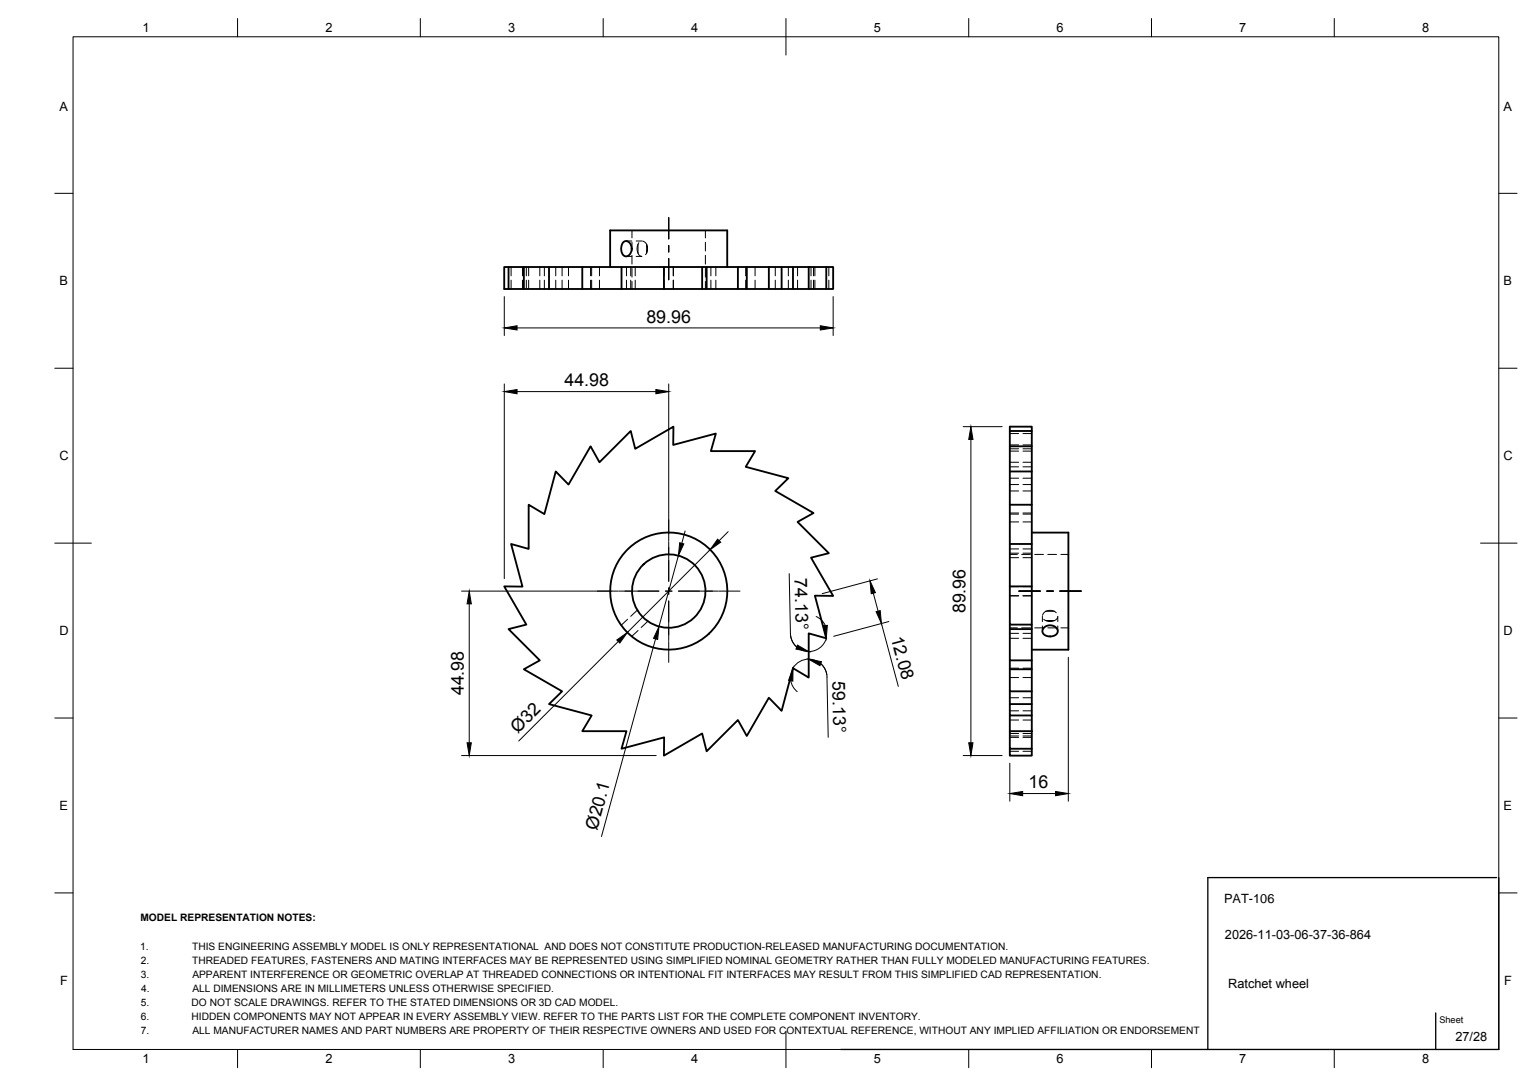
ISO-10303-21;
HEADER;
/* Generated by software containing ST-Developer
 * from STEP Tools, Inc. (www.steptools.com) 
 */

FILE_DESCRIPTION(
/* description */ ('Torsion-spring ratchet demonstrator'),
/* implementation_level */ '2;1');

FILE_NAME(
/* name */ 'Ratchet wheel.step',
/* time_stamp */ '2026-10-29T17:29:17-07:00',
/* author */ (''),
/* organization */ (''),
/* preprocessor_version */ 'ST-DEVELOPER v20.2',
/* originating_system */ 'Autodesk Translation Framework v15.17.0.0',
/* authorisation */ '');

FILE_SCHEMA (('AUTOMOTIVE_DESIGN { 1 0 10303 214 3 1 1 }'));
ENDSEC;

DATA;
#10=MECHANICAL_DESIGN_GEOMETRIC_PRESENTATION_REPRESENTATION('',(#312),#11258);
#231=B_SPLINE_CURVE_WITH_KNOTS('',3,(#10681,#10682,#10683,#10684,#10685,
#10686,#10687,#10688,#10689,#10690,#10691,#10692,#10693,#10694),
 .UNSPECIFIED.,.F.,.F.,(4,2,2,2,2,2,4),(0.75600573798702,0.793568827564647,
0.872922520054201,0.952276212543756,1.03162990503331,1.11098359752287,1.14854668710049),
 .UNSPECIFIED.);
#232=B_SPLINE_CURVE_WITH_KNOTS('',3,(#10700,#10701,#10702,#10703,#10704,
#10705,#10706,#10707,#10708,#10709,#10710,#10711,#10712,#10713,#10714,#10715,
#10716,#10717),.UNSPECIFIED.,.F.,.F.,(4,2,2,2,2,2,2,2,4),(0.,0.0792028026112439,
0.158405605222488,0.237607602356377,0.316809599490267,0.396011596624156,
0.475213593758045,0.554416396369289,0.633619198980533),.UNSPECIFIED.);
#233=B_SPLINE_CURVE_WITH_KNOTS('',3,(#10718,#10719,#10720,#10721,#10722,
#10723,#10724,#10725,#10726,#10727,#10728,#10729,#10730,#10731,#10732,#10733,
#10734,#10735),.UNSPECIFIED.,.F.,.F.,(4,2,2,2,2,2,2,2,4),(0.633619198980533,
0.712822001591777,0.792024804203021,0.87122680133691,0.950428798470799,
1.02963079560469,1.10883279273858,1.18803559534982,1.26723839796107),
 .UNSPECIFIED.);
#234=B_SPLINE_CURVE_WITH_KNOTS('',3,(#10738,#10739,#10740,#10741,#10742,
#10743,#10744,#10745,#10746,#10747,#10748,#10749,#10750,#10751),
 .UNSPECIFIED.,.F.,.F.,(4,2,2,2,2,2,4),(0.121154929624516,0.158718019202143,
0.238071711691697,0.317425404181252,0.396779096670807,0.476132789160362,
0.513695878737989),.UNSPECIFIED.);
#256=SHAPE_REPRESENTATION_RELATIONSHIP('SRR','None',#11384,#280);
#280=ADVANCED_BREP_SHAPE_REPRESENTATION('',(#342),#11254);
#312=STYLED_ITEM('',(#11577),#342);
#342=MANIFOLD_SOLID_BREP('Body1',#5185);
#429=FACE_BOUND('',#1237,.T.);
#430=FACE_BOUND('',#1239,.T.);
#431=FACE_BOUND('',#1241,.T.);
#432=FACE_BOUND('',#1291,.T.);
#433=FACE_BOUND('',#1293,.T.);
#549=PLANE('',#5948);
#550=PLANE('',#5953);
#551=PLANE('',#5957);
#552=PLANE('',#5961);
#553=PLANE('',#5962);
#554=PLANE('',#5963);
#555=PLANE('',#5964);
#556=PLANE('',#5965);
#557=PLANE('',#5966);
#558=PLANE('',#5967);
#559=PLANE('',#5968);
#560=PLANE('',#5969);
#561=PLANE('',#5970);
#562=PLANE('',#5971);
#563=PLANE('',#5972);
#564=PLANE('',#5973);
#565=PLANE('',#5974);
#566=PLANE('',#5975);
#567=PLANE('',#5976);
#568=PLANE('',#5977);
#569=PLANE('',#5978);
#570=PLANE('',#5979);
#571=PLANE('',#5980);
#572=PLANE('',#5981);
#573=PLANE('',#5982);
#574=PLANE('',#5983);
#575=PLANE('',#5984);
#576=PLANE('',#5985);
#577=PLANE('',#5986);
#578=PLANE('',#5987);
#579=PLANE('',#5988);
#580=PLANE('',#5989);
#581=PLANE('',#5990);
#582=PLANE('',#5991);
#583=PLANE('',#5992);
#584=PLANE('',#5993);
#585=PLANE('',#5994);
#586=PLANE('',#5995);
#587=PLANE('',#5996);
#588=PLANE('',#5997);
#589=PLANE('',#5998);
#590=PLANE('',#5999);
#591=PLANE('',#6000);
#592=PLANE('',#6001);
#593=PLANE('',#6002);
#594=PLANE('',#6003);
#595=PLANE('',#6004);
#596=PLANE('',#6005);
#597=PLANE('',#6006);
#598=PLANE('',#6007);
#599=PLANE('',#6008);
#600=PLANE('',#6009);
#601=PLANE('',#6010);
#844=FACE_OUTER_BOUND('',#1233,.T.);
#845=FACE_OUTER_BOUND('',#1234,.T.);
#846=FACE_OUTER_BOUND('',#1235,.T.);
#847=FACE_OUTER_BOUND('',#1236,.T.);
#848=FACE_OUTER_BOUND('',#1238,.T.);
#849=FACE_OUTER_BOUND('',#1240,.T.);
#850=FACE_OUTER_BOUND('',#1242,.T.);
#851=FACE_OUTER_BOUND('',#1243,.T.);
#852=FACE_OUTER_BOUND('',#1244,.T.);
#853=FACE_OUTER_BOUND('',#1245,.T.);
#854=FACE_OUTER_BOUND('',#1246,.T.);
#855=FACE_OUTER_BOUND('',#1247,.T.);
#856=FACE_OUTER_BOUND('',#1248,.T.);
#857=FACE_OUTER_BOUND('',#1249,.T.);
#858=FACE_OUTER_BOUND('',#1250,.T.);
#859=FACE_OUTER_BOUND('',#1251,.T.);
#860=FACE_OUTER_BOUND('',#1252,.T.);
#861=FACE_OUTER_BOUND('',#1253,.T.);
#862=FACE_OUTER_BOUND('',#1254,.T.);
#863=FACE_OUTER_BOUND('',#1255,.T.);
#864=FACE_OUTER_BOUND('',#1256,.T.);
#865=FACE_OUTER_BOUND('',#1257,.T.);
#866=FACE_OUTER_BOUND('',#1258,.T.);
#867=FACE_OUTER_BOUND('',#1259,.T.);
#868=FACE_OUTER_BOUND('',#1260,.T.);
#869=FACE_OUTER_BOUND('',#1261,.T.);
#870=FACE_OUTER_BOUND('',#1262,.T.);
#871=FACE_OUTER_BOUND('',#1263,.T.);
#872=FACE_OUTER_BOUND('',#1264,.T.);
#873=FACE_OUTER_BOUND('',#1265,.T.);
#874=FACE_OUTER_BOUND('',#1266,.T.);
#875=FACE_OUTER_BOUND('',#1267,.T.);
#876=FACE_OUTER_BOUND('',#1268,.T.);
#877=FACE_OUTER_BOUND('',#1269,.T.);
#878=FACE_OUTER_BOUND('',#1270,.T.);
#879=FACE_OUTER_BOUND('',#1271,.T.);
#880=FACE_OUTER_BOUND('',#1272,.T.);
#881=FACE_OUTER_BOUND('',#1273,.T.);
#882=FACE_OUTER_BOUND('',#1274,.T.);
#883=FACE_OUTER_BOUND('',#1275,.T.);
#884=FACE_OUTER_BOUND('',#1276,.T.);
#885=FACE_OUTER_BOUND('',#1277,.T.);
#886=FACE_OUTER_BOUND('',#1278,.T.);
#887=FACE_OUTER_BOUND('',#1279,.T.);
#888=FACE_OUTER_BOUND('',#1280,.T.);
#889=FACE_OUTER_BOUND('',#1281,.T.);
#890=FACE_OUTER_BOUND('',#1282,.T.);
#891=FACE_OUTER_BOUND('',#1283,.T.);
#892=FACE_OUTER_BOUND('',#1284,.T.);
#893=FACE_OUTER_BOUND('',#1285,.T.);
#894=FACE_OUTER_BOUND('',#1286,.T.);
#895=FACE_OUTER_BOUND('',#1287,.T.);
#896=FACE_OUTER_BOUND('',#1288,.T.);
#897=FACE_OUTER_BOUND('',#1289,.T.);
#898=FACE_OUTER_BOUND('',#1290,.T.);
#899=FACE_OUTER_BOUND('',#1292,.T.);
#1233=EDGE_LOOP('',(#4320,#4321));
#1234=EDGE_LOOP('',(#4322,#4323,#4324,#4325,#4326,#4327,#4328,#4329,#4330));
#1235=EDGE_LOOP('',(#4331,#4332,#4333));
#1236=EDGE_LOOP('',(#4334,#4335,#4336,#4337));
#1237=EDGE_LOOP('',(#4338,#4339));
#1238=EDGE_LOOP('',(#4340));
#1239=EDGE_LOOP('',(#4341));
#1240=EDGE_LOOP('',(#4342,#4343,#4344,#4345));
#1241=EDGE_LOOP('',(#4346,#4347,#4348,#4349));
#1242=EDGE_LOOP('',(#4350,#4351,#4352,#4353));
#1243=EDGE_LOOP('',(#4354,#4355,#4356,#4357));
#1244=EDGE_LOOP('',(#4358,#4359,#4360,#4361));
#1245=EDGE_LOOP('',(#4362,#4363,#4364,#4365));
#1246=EDGE_LOOP('',(#4366,#4367,#4368,#4369));
#1247=EDGE_LOOP('',(#4370,#4371,#4372,#4373));
#1248=EDGE_LOOP('',(#4374,#4375,#4376,#4377));
#1249=EDGE_LOOP('',(#4378,#4379,#4380,#4381));
#1250=EDGE_LOOP('',(#4382,#4383,#4384,#4385));
#1251=EDGE_LOOP('',(#4386,#4387,#4388,#4389));
#1252=EDGE_LOOP('',(#4390,#4391,#4392,#4393));
#1253=EDGE_LOOP('',(#4394,#4395,#4396,#4397));
#1254=EDGE_LOOP('',(#4398,#4399,#4400,#4401));
#1255=EDGE_LOOP('',(#4402,#4403,#4404,#4405));
#1256=EDGE_LOOP('',(#4406,#4407,#4408,#4409));
#1257=EDGE_LOOP('',(#4410,#4411,#4412,#4413));
#1258=EDGE_LOOP('',(#4414,#4415,#4416,#4417));
#1259=EDGE_LOOP('',(#4418,#4419,#4420,#4421));
#1260=EDGE_LOOP('',(#4422,#4423,#4424,#4425));
#1261=EDGE_LOOP('',(#4426,#4427,#4428,#4429));
#1262=EDGE_LOOP('',(#4430,#4431,#4432,#4433));
#1263=EDGE_LOOP('',(#4434,#4435,#4436,#4437));
#1264=EDGE_LOOP('',(#4438,#4439,#4440,#4441));
#1265=EDGE_LOOP('',(#4442,#4443,#4444,#4445));
#1266=EDGE_LOOP('',(#4446,#4447,#4448,#4449));
#1267=EDGE_LOOP('',(#4450,#4451,#4452,#4453));
#1268=EDGE_LOOP('',(#4454,#4455,#4456,#4457));
#1269=EDGE_LOOP('',(#4458,#4459,#4460,#4461));
#1270=EDGE_LOOP('',(#4462,#4463,#4464,#4465));
#1271=EDGE_LOOP('',(#4466,#4467,#4468,#4469));
#1272=EDGE_LOOP('',(#4470,#4471,#4472,#4473));
#1273=EDGE_LOOP('',(#4474,#4475,#4476,#4477));
#1274=EDGE_LOOP('',(#4478,#4479,#4480,#4481));
#1275=EDGE_LOOP('',(#4482,#4483,#4484,#4485));
#1276=EDGE_LOOP('',(#4486,#4487,#4488,#4489));
#1277=EDGE_LOOP('',(#4490,#4491,#4492,#4493));
#1278=EDGE_LOOP('',(#4494,#4495,#4496,#4497));
#1279=EDGE_LOOP('',(#4498,#4499,#4500,#4501));
#1280=EDGE_LOOP('',(#4502,#4503,#4504,#4505));
#1281=EDGE_LOOP('',(#4506,#4507,#4508,#4509));
#1282=EDGE_LOOP('',(#4510,#4511,#4512,#4513));
#1283=EDGE_LOOP('',(#4514,#4515,#4516,#4517));
#1284=EDGE_LOOP('',(#4518,#4519,#4520,#4521));
#1285=EDGE_LOOP('',(#4522,#4523,#4524,#4525));
#1286=EDGE_LOOP('',(#4526,#4527,#4528,#4529));
#1287=EDGE_LOOP('',(#4530,#4531,#4532,#4533));
#1288=EDGE_LOOP('',(#4534,#4535,#4536,#4537));
#1289=EDGE_LOOP('',(#4538,#4539,#4540,#4541));
#1290=EDGE_LOOP('',(#4542,#4543,#4544,#4545,#4546,#4547,#4548,#4549,#4550,
#4551,#4552,#4553,#4554,#4555,#4556,#4557,#4558,#4559,#4560,#4561,#4562,
#4563,#4564,#4565,#4566,#4567,#4568,#4569,#4570,#4571,#4572,#4573,#4574,
#4575,#4576,#4577,#4578,#4579,#4580,#4581,#4582,#4583,#4584,#4585,#4586,
#4587,#4588,#4589));
#1291=EDGE_LOOP('',(#4590));
#1292=EDGE_LOOP('',(#4591,#4592,#4593,#4594,#4595,#4596,#4597,#4598,#4599,
#4600,#4601,#4602,#4603,#4604,#4605,#4606,#4607,#4608,#4609,#4610,#4611,
#4612,#4613,#4614,#4615,#4616,#4617,#4618,#4619,#4620,#4621,#4622,#4623,
#4624,#4625,#4626,#4627,#4628,#4629,#4630,#4631,#4632,#4633,#4634,#4635,
#4636,#4637,#4638));
#1293=EDGE_LOOP('',(#4639));
#1511=LINE('',#10677,#1894);
#1512=LINE('',#10698,#1895);
#1513=LINE('',#10753,#1896);
#1514=LINE('',#10758,#1897);
#1515=LINE('',#10766,#1898);
#1516=LINE('',#10770,#1899);
#1517=LINE('',#10772,#1900);
#1518=LINE('',#10774,#1901);
#1519=LINE('',#10775,#1902);
#1520=LINE('',#10778,#1903);
#1521=LINE('',#10780,#1904);
#1522=LINE('',#10781,#1905);
#1523=LINE('',#10784,#1906);
#1524=LINE('',#10786,#1907);
#1525=LINE('',#10787,#1908);
#1526=LINE('',#10790,#1909);
#1527=LINE('',#10792,#1910);
#1528=LINE('',#10793,#1911);
#1529=LINE('',#10796,#1912);
#1530=LINE('',#10798,#1913);
#1531=LINE('',#10799,#1914);
#1532=LINE('',#10802,#1915);
#1533=LINE('',#10804,#1916);
#1534=LINE('',#10805,#1917);
#1535=LINE('',#10808,#1918);
#1536=LINE('',#10810,#1919);
#1537=LINE('',#10811,#1920);
#1538=LINE('',#10814,#1921);
#1539=LINE('',#10816,#1922);
#1540=LINE('',#10817,#1923);
#1541=LINE('',#10820,#1924);
#1542=LINE('',#10822,#1925);
#1543=LINE('',#10823,#1926);
#1544=LINE('',#10826,#1927);
#1545=LINE('',#10828,#1928);
#1546=LINE('',#10829,#1929);
#1547=LINE('',#10832,#1930);
#1548=LINE('',#10834,#1931);
#1549=LINE('',#10835,#1932);
#1550=LINE('',#10838,#1933);
#1551=LINE('',#10840,#1934);
#1552=LINE('',#10841,#1935);
#1553=LINE('',#10844,#1936);
#1554=LINE('',#10846,#1937);
#1555=LINE('',#10847,#1938);
#1556=LINE('',#10850,#1939);
#1557=LINE('',#10852,#1940);
#1558=LINE('',#10853,#1941);
#1559=LINE('',#10856,#1942);
#1560=LINE('',#10858,#1943);
#1561=LINE('',#10859,#1944);
#1562=LINE('',#10862,#1945);
#1563=LINE('',#10864,#1946);
#1564=LINE('',#10865,#1947);
#1565=LINE('',#10868,#1948);
#1566=LINE('',#10870,#1949);
#1567=LINE('',#10871,#1950);
#1568=LINE('',#10874,#1951);
#1569=LINE('',#10876,#1952);
#1570=LINE('',#10877,#1953);
#1571=LINE('',#10880,#1954);
#1572=LINE('',#10882,#1955);
#1573=LINE('',#10883,#1956);
#1574=LINE('',#10886,#1957);
#1575=LINE('',#10888,#1958);
#1576=LINE('',#10889,#1959);
#1577=LINE('',#10892,#1960);
#1578=LINE('',#10894,#1961);
#1579=LINE('',#10895,#1962);
#1580=LINE('',#10898,#1963);
#1581=LINE('',#10900,#1964);
#1582=LINE('',#10901,#1965);
#1583=LINE('',#10904,#1966);
#1584=LINE('',#10906,#1967);
#1585=LINE('',#10907,#1968);
#1586=LINE('',#10910,#1969);
#1587=LINE('',#10912,#1970);
#1588=LINE('',#10913,#1971);
#1589=LINE('',#10916,#1972);
#1590=LINE('',#10918,#1973);
#1591=LINE('',#10919,#1974);
#1592=LINE('',#10922,#1975);
#1593=LINE('',#10924,#1976);
#1594=LINE('',#10925,#1977);
#1595=LINE('',#10928,#1978);
#1596=LINE('',#10930,#1979);
#1597=LINE('',#10931,#1980);
#1598=LINE('',#10934,#1981);
#1599=LINE('',#10936,#1982);
#1600=LINE('',#10937,#1983);
#1601=LINE('',#10940,#1984);
#1602=LINE('',#10942,#1985);
#1603=LINE('',#10943,#1986);
#1604=LINE('',#10946,#1987);
#1605=LINE('',#10948,#1988);
#1606=LINE('',#10949,#1989);
#1607=LINE('',#10952,#1990);
#1608=LINE('',#10954,#1991);
#1609=LINE('',#10955,#1992);
#1610=LINE('',#10958,#1993);
#1611=LINE('',#10960,#1994);
#1612=LINE('',#10961,#1995);
#1613=LINE('',#10964,#1996);
#1614=LINE('',#10966,#1997);
#1615=LINE('',#10967,#1998);
#1616=LINE('',#10970,#1999);
#1617=LINE('',#10972,#2000);
#1618=LINE('',#10973,#2001);
#1619=LINE('',#10976,#2002);
#1620=LINE('',#10978,#2003);
#1621=LINE('',#10979,#2004);
#1622=LINE('',#10982,#2005);
#1623=LINE('',#10984,#2006);
#1624=LINE('',#10985,#2007);
#1625=LINE('',#10988,#2008);
#1626=LINE('',#10990,#2009);
#1627=LINE('',#10991,#2010);
#1628=LINE('',#10994,#2011);
#1629=LINE('',#10996,#2012);
#1630=LINE('',#10997,#2013);
#1631=LINE('',#11000,#2014);
#1632=LINE('',#11002,#2015);
#1633=LINE('',#11003,#2016);
#1634=LINE('',#11006,#2017);
#1635=LINE('',#11008,#2018);
#1636=LINE('',#11009,#2019);
#1637=LINE('',#11012,#2020);
#1638=LINE('',#11014,#2021);
#1639=LINE('',#11015,#2022);
#1640=LINE('',#11018,#2023);
#1641=LINE('',#11020,#2024);
#1642=LINE('',#11021,#2025);
#1643=LINE('',#11024,#2026);
#1644=LINE('',#11026,#2027);
#1645=LINE('',#11027,#2028);
#1646=LINE('',#11030,#2029);
#1647=LINE('',#11032,#2030);
#1648=LINE('',#11033,#2031);
#1649=LINE('',#11036,#2032);
#1650=LINE('',#11038,#2033);
#1651=LINE('',#11039,#2034);
#1652=LINE('',#11042,#2035);
#1653=LINE('',#11044,#2036);
#1654=LINE('',#11045,#2037);
#1655=LINE('',#11048,#2038);
#1656=LINE('',#11050,#2039);
#1657=LINE('',#11051,#2040);
#1658=LINE('',#11053,#2041);
#1659=LINE('',#11054,#2042);
#1894=VECTOR('',#7244,1.);
#1895=VECTOR('',#7251,0.21);
#1896=VECTOR('',#7256,1.);
#1897=VECTOR('',#7261,1.6);
#1898=VECTOR('',#7272,1.005);
#1899=VECTOR('',#7275,1.);
#1900=VECTOR('',#7276,1.);
#1901=VECTOR('',#7277,1.);
#1902=VECTOR('',#7278,1.);
#1903=VECTOR('',#7281,1.);
#1904=VECTOR('',#7282,1.);
#1905=VECTOR('',#7283,1.);
#1906=VECTOR('',#7286,1.);
#1907=VECTOR('',#7287,1.);
#1908=VECTOR('',#7288,1.);
#1909=VECTOR('',#7291,1.);
#1910=VECTOR('',#7292,1.);
#1911=VECTOR('',#7293,1.);
#1912=VECTOR('',#7296,1.);
#1913=VECTOR('',#7297,1.);
#1914=VECTOR('',#7298,1.);
#1915=VECTOR('',#7301,1.);
#1916=VECTOR('',#7302,1.);
#1917=VECTOR('',#7303,1.);
#1918=VECTOR('',#7306,1.);
#1919=VECTOR('',#7307,1.);
#1920=VECTOR('',#7308,1.);
#1921=VECTOR('',#7311,1.);
#1922=VECTOR('',#7312,1.);
#1923=VECTOR('',#7313,1.);
#1924=VECTOR('',#7316,1.);
#1925=VECTOR('',#7317,1.);
#1926=VECTOR('',#7318,1.);
#1927=VECTOR('',#7321,1.);
#1928=VECTOR('',#7322,1.);
#1929=VECTOR('',#7323,1.);
#1930=VECTOR('',#7326,1.);
#1931=VECTOR('',#7327,1.);
#1932=VECTOR('',#7328,1.);
#1933=VECTOR('',#7331,1.);
#1934=VECTOR('',#7332,1.);
#1935=VECTOR('',#7333,1.);
#1936=VECTOR('',#7336,1.);
#1937=VECTOR('',#7337,1.);
#1938=VECTOR('',#7338,1.);
#1939=VECTOR('',#7341,1.);
#1940=VECTOR('',#7342,1.);
#1941=VECTOR('',#7343,1.);
#1942=VECTOR('',#7346,1.);
#1943=VECTOR('',#7347,1.);
#1944=VECTOR('',#7348,1.);
#1945=VECTOR('',#7351,1.);
#1946=VECTOR('',#7352,1.);
#1947=VECTOR('',#7353,1.);
#1948=VECTOR('',#7356,1.);
#1949=VECTOR('',#7357,1.);
#1950=VECTOR('',#7358,1.);
#1951=VECTOR('',#7361,1.);
#1952=VECTOR('',#7362,1.);
#1953=VECTOR('',#7363,1.);
#1954=VECTOR('',#7366,1.);
#1955=VECTOR('',#7367,1.);
#1956=VECTOR('',#7368,1.);
#1957=VECTOR('',#7371,1.);
#1958=VECTOR('',#7372,1.);
#1959=VECTOR('',#7373,1.);
#1960=VECTOR('',#7376,1.);
#1961=VECTOR('',#7377,1.);
#1962=VECTOR('',#7378,1.);
#1963=VECTOR('',#7381,1.);
#1964=VECTOR('',#7382,1.);
#1965=VECTOR('',#7383,1.);
#1966=VECTOR('',#7386,1.);
#1967=VECTOR('',#7387,1.);
#1968=VECTOR('',#7388,1.);
#1969=VECTOR('',#7391,1.);
#1970=VECTOR('',#7392,1.);
#1971=VECTOR('',#7393,1.);
#1972=VECTOR('',#7396,1.);
#1973=VECTOR('',#7397,1.);
#1974=VECTOR('',#7398,1.);
#1975=VECTOR('',#7401,1.);
#1976=VECTOR('',#7402,1.);
#1977=VECTOR('',#7403,1.);
#1978=VECTOR('',#7406,1.);
#1979=VECTOR('',#7407,1.);
#1980=VECTOR('',#7408,1.);
#1981=VECTOR('',#7411,1.);
#1982=VECTOR('',#7412,1.);
#1983=VECTOR('',#7413,1.);
#1984=VECTOR('',#7416,1.);
#1985=VECTOR('',#7417,1.);
#1986=VECTOR('',#7418,1.);
#1987=VECTOR('',#7421,1.);
#1988=VECTOR('',#7422,1.);
#1989=VECTOR('',#7423,1.);
#1990=VECTOR('',#7426,1.);
#1991=VECTOR('',#7427,1.);
#1992=VECTOR('',#7428,1.);
#1993=VECTOR('',#7431,1.);
#1994=VECTOR('',#7432,1.);
#1995=VECTOR('',#7433,1.);
#1996=VECTOR('',#7436,1.);
#1997=VECTOR('',#7437,1.);
#1998=VECTOR('',#7438,1.);
#1999=VECTOR('',#7441,1.);
#2000=VECTOR('',#7442,1.);
#2001=VECTOR('',#7443,1.);
#2002=VECTOR('',#7446,1.);
#2003=VECTOR('',#7447,1.);
#2004=VECTOR('',#7448,1.);
#2005=VECTOR('',#7451,1.);
#2006=VECTOR('',#7452,1.);
#2007=VECTOR('',#7453,1.);
#2008=VECTOR('',#7456,1.);
#2009=VECTOR('',#7457,1.);
#2010=VECTOR('',#7458,1.);
#2011=VECTOR('',#7461,1.);
#2012=VECTOR('',#7462,1.);
#2013=VECTOR('',#7463,1.);
#2014=VECTOR('',#7466,1.);
#2015=VECTOR('',#7467,1.);
#2016=VECTOR('',#7468,1.);
#2017=VECTOR('',#7471,1.);
#2018=VECTOR('',#7472,1.);
#2019=VECTOR('',#7473,1.);
#2020=VECTOR('',#7476,1.);
#2021=VECTOR('',#7477,1.);
#2022=VECTOR('',#7478,1.);
#2023=VECTOR('',#7481,1.);
#2024=VECTOR('',#7482,1.);
#2025=VECTOR('',#7483,1.);
#2026=VECTOR('',#7486,1.);
#2027=VECTOR('',#7487,1.);
#2028=VECTOR('',#7488,1.);
#2029=VECTOR('',#7491,1.);
#2030=VECTOR('',#7492,1.);
#2031=VECTOR('',#7493,1.);
#2032=VECTOR('',#7496,1.);
#2033=VECTOR('',#7497,1.);
#2034=VECTOR('',#7498,1.);
#2035=VECTOR('',#7501,1.);
#2036=VECTOR('',#7502,1.);
#2037=VECTOR('',#7503,1.);
#2038=VECTOR('',#7506,1.);
#2039=VECTOR('',#7507,1.);
#2040=VECTOR('',#7508,1.);
#2041=VECTOR('',#7511,1.);
#2042=VECTOR('',#7512,1.);
#2314=CIRCLE('',#5949,0.21);
#2315=CIRCLE('',#5951,0.21);
#2316=CIRCLE('',#5952,0.21);
#2317=CIRCLE('',#5955,1.6);
#2318=CIRCLE('',#5956,1.6);
#2319=CIRCLE('',#5958,1.005);
#2320=CIRCLE('',#5960,1.005);
#2635=VERTEX_POINT('',#10675);
#2636=VERTEX_POINT('',#10676);
#2637=VERTEX_POINT('',#10680);
#2638=VERTEX_POINT('',#10695);
#2639=VERTEX_POINT('',#10697);
#2640=VERTEX_POINT('',#10699);
#2641=VERTEX_POINT('',#10736);
#2642=VERTEX_POINT('',#10755);
#2643=VERTEX_POINT('',#10757);
#2644=VERTEX_POINT('',#10761);
#2645=VERTEX_POINT('',#10764);
#2646=VERTEX_POINT('',#10768);
#2647=VERTEX_POINT('',#10769);
#2648=VERTEX_POINT('',#10771);
#2649=VERTEX_POINT('',#10773);
#2650=VERTEX_POINT('',#10777);
#2651=VERTEX_POINT('',#10779);
#2652=VERTEX_POINT('',#10783);
#2653=VERTEX_POINT('',#10785);
#2654=VERTEX_POINT('',#10789);
#2655=VERTEX_POINT('',#10791);
#2656=VERTEX_POINT('',#10795);
#2657=VERTEX_POINT('',#10797);
#2658=VERTEX_POINT('',#10801);
#2659=VERTEX_POINT('',#10803);
#2660=VERTEX_POINT('',#10807);
#2661=VERTEX_POINT('',#10809);
#2662=VERTEX_POINT('',#10813);
#2663=VERTEX_POINT('',#10815);
#2664=VERTEX_POINT('',#10819);
#2665=VERTEX_POINT('',#10821);
#2666=VERTEX_POINT('',#10825);
#2667=VERTEX_POINT('',#10827);
#2668=VERTEX_POINT('',#10831);
#2669=VERTEX_POINT('',#10833);
#2670=VERTEX_POINT('',#10837);
#2671=VERTEX_POINT('',#10839);
#2672=VERTEX_POINT('',#10843);
#2673=VERTEX_POINT('',#10845);
#2674=VERTEX_POINT('',#10849);
#2675=VERTEX_POINT('',#10851);
#2676=VERTEX_POINT('',#10855);
#2677=VERTEX_POINT('',#10857);
#2678=VERTEX_POINT('',#10861);
#2679=VERTEX_POINT('',#10863);
#2680=VERTEX_POINT('',#10867);
#2681=VERTEX_POINT('',#10869);
#2682=VERTEX_POINT('',#10873);
#2683=VERTEX_POINT('',#10875);
#2684=VERTEX_POINT('',#10879);
#2685=VERTEX_POINT('',#10881);
#2686=VERTEX_POINT('',#10885);
#2687=VERTEX_POINT('',#10887);
#2688=VERTEX_POINT('',#10891);
#2689=VERTEX_POINT('',#10893);
#2690=VERTEX_POINT('',#10897);
#2691=VERTEX_POINT('',#10899);
#2692=VERTEX_POINT('',#10903);
#2693=VERTEX_POINT('',#10905);
#2694=VERTEX_POINT('',#10909);
#2695=VERTEX_POINT('',#10911);
#2696=VERTEX_POINT('',#10915);
#2697=VERTEX_POINT('',#10917);
#2698=VERTEX_POINT('',#10921);
#2699=VERTEX_POINT('',#10923);
#2700=VERTEX_POINT('',#10927);
#2701=VERTEX_POINT('',#10929);
#2702=VERTEX_POINT('',#10933);
#2703=VERTEX_POINT('',#10935);
#2704=VERTEX_POINT('',#10939);
#2705=VERTEX_POINT('',#10941);
#2706=VERTEX_POINT('',#10945);
#2707=VERTEX_POINT('',#10947);
#2708=VERTEX_POINT('',#10951);
#2709=VERTEX_POINT('',#10953);
#2710=VERTEX_POINT('',#10957);
#2711=VERTEX_POINT('',#10959);
#2712=VERTEX_POINT('',#10963);
#2713=VERTEX_POINT('',#10965);
#2714=VERTEX_POINT('',#10969);
#2715=VERTEX_POINT('',#10971);
#2716=VERTEX_POINT('',#10975);
#2717=VERTEX_POINT('',#10977);
#2718=VERTEX_POINT('',#10981);
#2719=VERTEX_POINT('',#10983);
#2720=VERTEX_POINT('',#10987);
#2721=VERTEX_POINT('',#10989);
#2722=VERTEX_POINT('',#10993);
#2723=VERTEX_POINT('',#10995);
#2724=VERTEX_POINT('',#10999);
#2725=VERTEX_POINT('',#11001);
#2726=VERTEX_POINT('',#11005);
#2727=VERTEX_POINT('',#11007);
#2728=VERTEX_POINT('',#11011);
#2729=VERTEX_POINT('',#11013);
#2730=VERTEX_POINT('',#11017);
#2731=VERTEX_POINT('',#11019);
#2732=VERTEX_POINT('',#11023);
#2733=VERTEX_POINT('',#11025);
#2734=VERTEX_POINT('',#11029);
#2735=VERTEX_POINT('',#11031);
#2736=VERTEX_POINT('',#11035);
#2737=VERTEX_POINT('',#11037);
#2738=VERTEX_POINT('',#11041);
#2739=VERTEX_POINT('',#11043);
#2740=VERTEX_POINT('',#11047);
#2741=VERTEX_POINT('',#11049);
#3220=EDGE_CURVE('',#2635,#2636,#1511,.T.);
#3221=EDGE_CURVE('',#2635,#2636,#2314,.T.);
#3222=EDGE_CURVE('',#2637,#2635,#231,.T.);
#3223=EDGE_CURVE('',#2638,#2637,#2315,.T.);
#3224=EDGE_CURVE('',#2638,#2639,#1512,.T.);
#3225=EDGE_CURVE('',#2640,#2639,#232,.T.);
#3226=EDGE_CURVE('',#2639,#2640,#233,.T.);
#3227=EDGE_CURVE('',#2641,#2638,#2316,.T.);
#3228=EDGE_CURVE('',#2636,#2641,#234,.T.);
#3229=EDGE_CURVE('',#2641,#2637,#1513,.T.);
#3230=EDGE_CURVE('',#2642,#2642,#2317,.T.);
#3231=EDGE_CURVE('',#2642,#2643,#1514,.T.);
#3232=EDGE_CURVE('',#2643,#2643,#2318,.T.);
#3233=EDGE_CURVE('',#2644,#2644,#2319,.T.);
#3234=EDGE_CURVE('',#2645,#2645,#2320,.T.);
#3235=EDGE_CURVE('',#2645,#2644,#1515,.T.);
#3236=EDGE_CURVE('',#2646,#2647,#1516,.T.);
#3237=EDGE_CURVE('',#2646,#2648,#1517,.T.);
#3238=EDGE_CURVE('',#2649,#2648,#1518,.T.);
#3239=EDGE_CURVE('',#2647,#2649,#1519,.T.);
#3240=EDGE_CURVE('',#2647,#2650,#1520,.T.);
#3241=EDGE_CURVE('',#2651,#2649,#1521,.T.);
#3242=EDGE_CURVE('',#2650,#2651,#1522,.T.);
#3243=EDGE_CURVE('',#2650,#2652,#1523,.T.);
#3244=EDGE_CURVE('',#2653,#2651,#1524,.T.);
#3245=EDGE_CURVE('',#2652,#2653,#1525,.T.);
#3246=EDGE_CURVE('',#2652,#2654,#1526,.T.);
#3247=EDGE_CURVE('',#2655,#2653,#1527,.T.);
#3248=EDGE_CURVE('',#2654,#2655,#1528,.T.);
#3249=EDGE_CURVE('',#2654,#2656,#1529,.T.);
#3250=EDGE_CURVE('',#2657,#2655,#1530,.T.);
#3251=EDGE_CURVE('',#2656,#2657,#1531,.T.);
#3252=EDGE_CURVE('',#2656,#2658,#1532,.T.);
#3253=EDGE_CURVE('',#2659,#2657,#1533,.T.);
#3254=EDGE_CURVE('',#2658,#2659,#1534,.T.);
#3255=EDGE_CURVE('',#2658,#2660,#1535,.T.);
#3256=EDGE_CURVE('',#2661,#2659,#1536,.T.);
#3257=EDGE_CURVE('',#2660,#2661,#1537,.T.);
#3258=EDGE_CURVE('',#2660,#2662,#1538,.T.);
#3259=EDGE_CURVE('',#2663,#2661,#1539,.T.);
#3260=EDGE_CURVE('',#2662,#2663,#1540,.T.);
#3261=EDGE_CURVE('',#2662,#2664,#1541,.T.);
#3262=EDGE_CURVE('',#2665,#2663,#1542,.T.);
#3263=EDGE_CURVE('',#2664,#2665,#1543,.T.);
#3264=EDGE_CURVE('',#2664,#2666,#1544,.T.);
#3265=EDGE_CURVE('',#2667,#2665,#1545,.T.);
#3266=EDGE_CURVE('',#2666,#2667,#1546,.T.);
#3267=EDGE_CURVE('',#2666,#2668,#1547,.T.);
#3268=EDGE_CURVE('',#2669,#2667,#1548,.T.);
#3269=EDGE_CURVE('',#2668,#2669,#1549,.T.);
#3270=EDGE_CURVE('',#2668,#2670,#1550,.T.);
#3271=EDGE_CURVE('',#2671,#2669,#1551,.T.);
#3272=EDGE_CURVE('',#2670,#2671,#1552,.T.);
#3273=EDGE_CURVE('',#2670,#2672,#1553,.T.);
#3274=EDGE_CURVE('',#2673,#2671,#1554,.T.);
#3275=EDGE_CURVE('',#2672,#2673,#1555,.T.);
#3276=EDGE_CURVE('',#2672,#2674,#1556,.T.);
#3277=EDGE_CURVE('',#2675,#2673,#1557,.T.);
#3278=EDGE_CURVE('',#2674,#2675,#1558,.T.);
#3279=EDGE_CURVE('',#2674,#2676,#1559,.T.);
#3280=EDGE_CURVE('',#2677,#2675,#1560,.T.);
#3281=EDGE_CURVE('',#2676,#2677,#1561,.T.);
#3282=EDGE_CURVE('',#2676,#2678,#1562,.T.);
#3283=EDGE_CURVE('',#2679,#2677,#1563,.T.);
#3284=EDGE_CURVE('',#2678,#2679,#1564,.T.);
#3285=EDGE_CURVE('',#2678,#2680,#1565,.T.);
#3286=EDGE_CURVE('',#2681,#2679,#1566,.T.);
#3287=EDGE_CURVE('',#2680,#2681,#1567,.T.);
#3288=EDGE_CURVE('',#2680,#2682,#1568,.T.);
#3289=EDGE_CURVE('',#2683,#2681,#1569,.T.);
#3290=EDGE_CURVE('',#2682,#2683,#1570,.T.);
#3291=EDGE_CURVE('',#2682,#2684,#1571,.T.);
#3292=EDGE_CURVE('',#2685,#2683,#1572,.T.);
#3293=EDGE_CURVE('',#2684,#2685,#1573,.T.);
#3294=EDGE_CURVE('',#2684,#2686,#1574,.T.);
#3295=EDGE_CURVE('',#2687,#2685,#1575,.T.);
#3296=EDGE_CURVE('',#2686,#2687,#1576,.T.);
#3297=EDGE_CURVE('',#2686,#2688,#1577,.T.);
#3298=EDGE_CURVE('',#2689,#2687,#1578,.T.);
#3299=EDGE_CURVE('',#2688,#2689,#1579,.T.);
#3300=EDGE_CURVE('',#2688,#2690,#1580,.T.);
#3301=EDGE_CURVE('',#2691,#2689,#1581,.T.);
#3302=EDGE_CURVE('',#2690,#2691,#1582,.T.);
#3303=EDGE_CURVE('',#2690,#2692,#1583,.T.);
#3304=EDGE_CURVE('',#2693,#2691,#1584,.T.);
#3305=EDGE_CURVE('',#2692,#2693,#1585,.T.);
#3306=EDGE_CURVE('',#2692,#2694,#1586,.T.);
#3307=EDGE_CURVE('',#2695,#2693,#1587,.T.);
#3308=EDGE_CURVE('',#2694,#2695,#1588,.T.);
#3309=EDGE_CURVE('',#2694,#2696,#1589,.T.);
#3310=EDGE_CURVE('',#2697,#2695,#1590,.T.);
#3311=EDGE_CURVE('',#2696,#2697,#1591,.T.);
#3312=EDGE_CURVE('',#2696,#2698,#1592,.T.);
#3313=EDGE_CURVE('',#2699,#2697,#1593,.T.);
#3314=EDGE_CURVE('',#2698,#2699,#1594,.T.);
#3315=EDGE_CURVE('',#2698,#2700,#1595,.T.);
#3316=EDGE_CURVE('',#2701,#2699,#1596,.T.);
#3317=EDGE_CURVE('',#2700,#2701,#1597,.T.);
#3318=EDGE_CURVE('',#2700,#2702,#1598,.T.);
#3319=EDGE_CURVE('',#2703,#2701,#1599,.T.);
#3320=EDGE_CURVE('',#2702,#2703,#1600,.T.);
#3321=EDGE_CURVE('',#2702,#2704,#1601,.T.);
#3322=EDGE_CURVE('',#2705,#2703,#1602,.T.);
#3323=EDGE_CURVE('',#2704,#2705,#1603,.T.);
#3324=EDGE_CURVE('',#2704,#2706,#1604,.T.);
#3325=EDGE_CURVE('',#2707,#2705,#1605,.T.);
#3326=EDGE_CURVE('',#2706,#2707,#1606,.T.);
#3327=EDGE_CURVE('',#2706,#2708,#1607,.T.);
#3328=EDGE_CURVE('',#2709,#2707,#1608,.T.);
#3329=EDGE_CURVE('',#2708,#2709,#1609,.T.);
#3330=EDGE_CURVE('',#2708,#2710,#1610,.T.);
#3331=EDGE_CURVE('',#2711,#2709,#1611,.T.);
#3332=EDGE_CURVE('',#2710,#2711,#1612,.T.);
#3333=EDGE_CURVE('',#2710,#2712,#1613,.T.);
#3334=EDGE_CURVE('',#2713,#2711,#1614,.T.);
#3335=EDGE_CURVE('',#2712,#2713,#1615,.T.);
#3336=EDGE_CURVE('',#2712,#2714,#1616,.T.);
#3337=EDGE_CURVE('',#2715,#2713,#1617,.T.);
#3338=EDGE_CURVE('',#2714,#2715,#1618,.T.);
#3339=EDGE_CURVE('',#2714,#2716,#1619,.T.);
#3340=EDGE_CURVE('',#2717,#2715,#1620,.T.);
#3341=EDGE_CURVE('',#2716,#2717,#1621,.T.);
#3342=EDGE_CURVE('',#2716,#2718,#1622,.T.);
#3343=EDGE_CURVE('',#2719,#2717,#1623,.T.);
#3344=EDGE_CURVE('',#2718,#2719,#1624,.T.);
#3345=EDGE_CURVE('',#2718,#2720,#1625,.T.);
#3346=EDGE_CURVE('',#2721,#2719,#1626,.T.);
#3347=EDGE_CURVE('',#2720,#2721,#1627,.T.);
#3348=EDGE_CURVE('',#2720,#2722,#1628,.T.);
#3349=EDGE_CURVE('',#2723,#2721,#1629,.T.);
#3350=EDGE_CURVE('',#2722,#2723,#1630,.T.);
#3351=EDGE_CURVE('',#2722,#2724,#1631,.T.);
#3352=EDGE_CURVE('',#2725,#2723,#1632,.T.);
#3353=EDGE_CURVE('',#2724,#2725,#1633,.T.);
#3354=EDGE_CURVE('',#2724,#2726,#1634,.T.);
#3355=EDGE_CURVE('',#2727,#2725,#1635,.T.);
#3356=EDGE_CURVE('',#2726,#2727,#1636,.T.);
#3357=EDGE_CURVE('',#2726,#2728,#1637,.T.);
#3358=EDGE_CURVE('',#2729,#2727,#1638,.T.);
#3359=EDGE_CURVE('',#2728,#2729,#1639,.T.);
#3360=EDGE_CURVE('',#2728,#2730,#1640,.T.);
#3361=EDGE_CURVE('',#2731,#2729,#1641,.T.);
#3362=EDGE_CURVE('',#2730,#2731,#1642,.T.);
#3363=EDGE_CURVE('',#2730,#2732,#1643,.T.);
#3364=EDGE_CURVE('',#2733,#2731,#1644,.T.);
#3365=EDGE_CURVE('',#2732,#2733,#1645,.T.);
#3366=EDGE_CURVE('',#2732,#2734,#1646,.T.);
#3367=EDGE_CURVE('',#2735,#2733,#1647,.T.);
#3368=EDGE_CURVE('',#2734,#2735,#1648,.T.);
#3369=EDGE_CURVE('',#2734,#2736,#1649,.T.);
#3370=EDGE_CURVE('',#2737,#2735,#1650,.T.);
#3371=EDGE_CURVE('',#2736,#2737,#1651,.T.);
#3372=EDGE_CURVE('',#2736,#2738,#1652,.T.);
#3373=EDGE_CURVE('',#2739,#2737,#1653,.T.);
#3374=EDGE_CURVE('',#2738,#2739,#1654,.T.);
#3375=EDGE_CURVE('',#2738,#2740,#1655,.T.);
#3376=EDGE_CURVE('',#2741,#2739,#1656,.T.);
#3377=EDGE_CURVE('',#2740,#2741,#1657,.T.);
#3378=EDGE_CURVE('',#2740,#2646,#1658,.T.);
#3379=EDGE_CURVE('',#2648,#2741,#1659,.T.);
#4320=ORIENTED_EDGE('',*,*,#3220,.F.);
#4321=ORIENTED_EDGE('',*,*,#3221,.T.);
#4322=ORIENTED_EDGE('',*,*,#3222,.F.);
#4323=ORIENTED_EDGE('',*,*,#3223,.F.);
#4324=ORIENTED_EDGE('',*,*,#3224,.T.);
#4325=ORIENTED_EDGE('',*,*,#3225,.F.);
#4326=ORIENTED_EDGE('',*,*,#3226,.F.);
#4327=ORIENTED_EDGE('',*,*,#3224,.F.);
#4328=ORIENTED_EDGE('',*,*,#3227,.F.);
#4329=ORIENTED_EDGE('',*,*,#3228,.F.);
#4330=ORIENTED_EDGE('',*,*,#3221,.F.);
#4331=ORIENTED_EDGE('',*,*,#3229,.F.);
#4332=ORIENTED_EDGE('',*,*,#3227,.T.);
#4333=ORIENTED_EDGE('',*,*,#3223,.T.);
#4334=ORIENTED_EDGE('',*,*,#3230,.F.);
#4335=ORIENTED_EDGE('',*,*,#3231,.T.);
#4336=ORIENTED_EDGE('',*,*,#3232,.F.);
#4337=ORIENTED_EDGE('',*,*,#3231,.F.);
#4338=ORIENTED_EDGE('',*,*,#3225,.T.);
#4339=ORIENTED_EDGE('',*,*,#3226,.T.);
#4340=ORIENTED_EDGE('',*,*,#3230,.T.);
#4341=ORIENTED_EDGE('',*,*,#3233,.T.);
#4342=ORIENTED_EDGE('',*,*,#3234,.F.);
#4343=ORIENTED_EDGE('',*,*,#3235,.T.);
#4344=ORIENTED_EDGE('',*,*,#3233,.F.);
#4345=ORIENTED_EDGE('',*,*,#3235,.F.);
#4346=ORIENTED_EDGE('',*,*,#3228,.T.);
#4347=ORIENTED_EDGE('',*,*,#3229,.T.);
#4348=ORIENTED_EDGE('',*,*,#3222,.T.);
#4349=ORIENTED_EDGE('',*,*,#3220,.T.);
#4350=ORIENTED_EDGE('',*,*,#3236,.F.);
#4351=ORIENTED_EDGE('',*,*,#3237,.T.);
#4352=ORIENTED_EDGE('',*,*,#3238,.F.);
#4353=ORIENTED_EDGE('',*,*,#3239,.F.);
#4354=ORIENTED_EDGE('',*,*,#3240,.F.);
#4355=ORIENTED_EDGE('',*,*,#3239,.T.);
#4356=ORIENTED_EDGE('',*,*,#3241,.F.);
#4357=ORIENTED_EDGE('',*,*,#3242,.F.);
#4358=ORIENTED_EDGE('',*,*,#3243,.F.);
#4359=ORIENTED_EDGE('',*,*,#3242,.T.);
#4360=ORIENTED_EDGE('',*,*,#3244,.F.);
#4361=ORIENTED_EDGE('',*,*,#3245,.F.);
#4362=ORIENTED_EDGE('',*,*,#3246,.F.);
#4363=ORIENTED_EDGE('',*,*,#3245,.T.);
#4364=ORIENTED_EDGE('',*,*,#3247,.F.);
#4365=ORIENTED_EDGE('',*,*,#3248,.F.);
#4366=ORIENTED_EDGE('',*,*,#3249,.F.);
#4367=ORIENTED_EDGE('',*,*,#3248,.T.);
#4368=ORIENTED_EDGE('',*,*,#3250,.F.);
#4369=ORIENTED_EDGE('',*,*,#3251,.F.);
#4370=ORIENTED_EDGE('',*,*,#3252,.F.);
#4371=ORIENTED_EDGE('',*,*,#3251,.T.);
#4372=ORIENTED_EDGE('',*,*,#3253,.F.);
#4373=ORIENTED_EDGE('',*,*,#3254,.F.);
#4374=ORIENTED_EDGE('',*,*,#3255,.F.);
#4375=ORIENTED_EDGE('',*,*,#3254,.T.);
#4376=ORIENTED_EDGE('',*,*,#3256,.F.);
#4377=ORIENTED_EDGE('',*,*,#3257,.F.);
#4378=ORIENTED_EDGE('',*,*,#3258,.F.);
#4379=ORIENTED_EDGE('',*,*,#3257,.T.);
#4380=ORIENTED_EDGE('',*,*,#3259,.F.);
#4381=ORIENTED_EDGE('',*,*,#3260,.F.);
#4382=ORIENTED_EDGE('',*,*,#3261,.F.);
#4383=ORIENTED_EDGE('',*,*,#3260,.T.);
#4384=ORIENTED_EDGE('',*,*,#3262,.F.);
#4385=ORIENTED_EDGE('',*,*,#3263,.F.);
#4386=ORIENTED_EDGE('',*,*,#3264,.F.);
#4387=ORIENTED_EDGE('',*,*,#3263,.T.);
#4388=ORIENTED_EDGE('',*,*,#3265,.F.);
#4389=ORIENTED_EDGE('',*,*,#3266,.F.);
#4390=ORIENTED_EDGE('',*,*,#3267,.F.);
#4391=ORIENTED_EDGE('',*,*,#3266,.T.);
#4392=ORIENTED_EDGE('',*,*,#3268,.F.);
#4393=ORIENTED_EDGE('',*,*,#3269,.F.);
#4394=ORIENTED_EDGE('',*,*,#3270,.F.);
#4395=ORIENTED_EDGE('',*,*,#3269,.T.);
#4396=ORIENTED_EDGE('',*,*,#3271,.F.);
#4397=ORIENTED_EDGE('',*,*,#3272,.F.);
#4398=ORIENTED_EDGE('',*,*,#3273,.F.);
#4399=ORIENTED_EDGE('',*,*,#3272,.T.);
#4400=ORIENTED_EDGE('',*,*,#3274,.F.);
#4401=ORIENTED_EDGE('',*,*,#3275,.F.);
#4402=ORIENTED_EDGE('',*,*,#3276,.F.);
#4403=ORIENTED_EDGE('',*,*,#3275,.T.);
#4404=ORIENTED_EDGE('',*,*,#3277,.F.);
#4405=ORIENTED_EDGE('',*,*,#3278,.F.);
#4406=ORIENTED_EDGE('',*,*,#3279,.F.);
#4407=ORIENTED_EDGE('',*,*,#3278,.T.);
#4408=ORIENTED_EDGE('',*,*,#3280,.F.);
#4409=ORIENTED_EDGE('',*,*,#3281,.F.);
#4410=ORIENTED_EDGE('',*,*,#3282,.F.);
#4411=ORIENTED_EDGE('',*,*,#3281,.T.);
#4412=ORIENTED_EDGE('',*,*,#3283,.F.);
#4413=ORIENTED_EDGE('',*,*,#3284,.F.);
#4414=ORIENTED_EDGE('',*,*,#3285,.F.);
#4415=ORIENTED_EDGE('',*,*,#3284,.T.);
#4416=ORIENTED_EDGE('',*,*,#3286,.F.);
#4417=ORIENTED_EDGE('',*,*,#3287,.F.);
#4418=ORIENTED_EDGE('',*,*,#3288,.F.);
#4419=ORIENTED_EDGE('',*,*,#3287,.T.);
#4420=ORIENTED_EDGE('',*,*,#3289,.F.);
#4421=ORIENTED_EDGE('',*,*,#3290,.F.);
#4422=ORIENTED_EDGE('',*,*,#3291,.F.);
#4423=ORIENTED_EDGE('',*,*,#3290,.T.);
#4424=ORIENTED_EDGE('',*,*,#3292,.F.);
#4425=ORIENTED_EDGE('',*,*,#3293,.F.);
#4426=ORIENTED_EDGE('',*,*,#3294,.F.);
#4427=ORIENTED_EDGE('',*,*,#3293,.T.);
#4428=ORIENTED_EDGE('',*,*,#3295,.F.);
#4429=ORIENTED_EDGE('',*,*,#3296,.F.);
#4430=ORIENTED_EDGE('',*,*,#3297,.F.);
#4431=ORIENTED_EDGE('',*,*,#3296,.T.);
#4432=ORIENTED_EDGE('',*,*,#3298,.F.);
#4433=ORIENTED_EDGE('',*,*,#3299,.F.);
#4434=ORIENTED_EDGE('',*,*,#3300,.F.);
#4435=ORIENTED_EDGE('',*,*,#3299,.T.);
#4436=ORIENTED_EDGE('',*,*,#3301,.F.);
#4437=ORIENTED_EDGE('',*,*,#3302,.F.);
#4438=ORIENTED_EDGE('',*,*,#3303,.F.);
#4439=ORIENTED_EDGE('',*,*,#3302,.T.);
#4440=ORIENTED_EDGE('',*,*,#3304,.F.);
#4441=ORIENTED_EDGE('',*,*,#3305,.F.);
#4442=ORIENTED_EDGE('',*,*,#3306,.F.);
#4443=ORIENTED_EDGE('',*,*,#3305,.T.);
#4444=ORIENTED_EDGE('',*,*,#3307,.F.);
#4445=ORIENTED_EDGE('',*,*,#3308,.F.);
#4446=ORIENTED_EDGE('',*,*,#3309,.F.);
#4447=ORIENTED_EDGE('',*,*,#3308,.T.);
#4448=ORIENTED_EDGE('',*,*,#3310,.F.);
#4449=ORIENTED_EDGE('',*,*,#3311,.F.);
#4450=ORIENTED_EDGE('',*,*,#3312,.F.);
#4451=ORIENTED_EDGE('',*,*,#3311,.T.);
#4452=ORIENTED_EDGE('',*,*,#3313,.F.);
#4453=ORIENTED_EDGE('',*,*,#3314,.F.);
#4454=ORIENTED_EDGE('',*,*,#3315,.F.);
#4455=ORIENTED_EDGE('',*,*,#3314,.T.);
#4456=ORIENTED_EDGE('',*,*,#3316,.F.);
#4457=ORIENTED_EDGE('',*,*,#3317,.F.);
#4458=ORIENTED_EDGE('',*,*,#3318,.F.);
#4459=ORIENTED_EDGE('',*,*,#3317,.T.);
#4460=ORIENTED_EDGE('',*,*,#3319,.F.);
#4461=ORIENTED_EDGE('',*,*,#3320,.F.);
#4462=ORIENTED_EDGE('',*,*,#3321,.F.);
#4463=ORIENTED_EDGE('',*,*,#3320,.T.);
#4464=ORIENTED_EDGE('',*,*,#3322,.F.);
#4465=ORIENTED_EDGE('',*,*,#3323,.F.);
#4466=ORIENTED_EDGE('',*,*,#3324,.F.);
#4467=ORIENTED_EDGE('',*,*,#3323,.T.);
#4468=ORIENTED_EDGE('',*,*,#3325,.F.);
#4469=ORIENTED_EDGE('',*,*,#3326,.F.);
#4470=ORIENTED_EDGE('',*,*,#3327,.F.);
#4471=ORIENTED_EDGE('',*,*,#3326,.T.);
#4472=ORIENTED_EDGE('',*,*,#3328,.F.);
#4473=ORIENTED_EDGE('',*,*,#3329,.F.);
#4474=ORIENTED_EDGE('',*,*,#3330,.F.);
#4475=ORIENTED_EDGE('',*,*,#3329,.T.);
#4476=ORIENTED_EDGE('',*,*,#3331,.F.);
#4477=ORIENTED_EDGE('',*,*,#3332,.F.);
#4478=ORIENTED_EDGE('',*,*,#3333,.F.);
#4479=ORIENTED_EDGE('',*,*,#3332,.T.);
#4480=ORIENTED_EDGE('',*,*,#3334,.F.);
#4481=ORIENTED_EDGE('',*,*,#3335,.F.);
#4482=ORIENTED_EDGE('',*,*,#3336,.F.);
#4483=ORIENTED_EDGE('',*,*,#3335,.T.);
#4484=ORIENTED_EDGE('',*,*,#3337,.F.);
#4485=ORIENTED_EDGE('',*,*,#3338,.F.);
#4486=ORIENTED_EDGE('',*,*,#3339,.F.);
#4487=ORIENTED_EDGE('',*,*,#3338,.T.);
#4488=ORIENTED_EDGE('',*,*,#3340,.F.);
#4489=ORIENTED_EDGE('',*,*,#3341,.F.);
#4490=ORIENTED_EDGE('',*,*,#3342,.F.);
#4491=ORIENTED_EDGE('',*,*,#3341,.T.);
#4492=ORIENTED_EDGE('',*,*,#3343,.F.);
#4493=ORIENTED_EDGE('',*,*,#3344,.F.);
#4494=ORIENTED_EDGE('',*,*,#3345,.F.);
#4495=ORIENTED_EDGE('',*,*,#3344,.T.);
#4496=ORIENTED_EDGE('',*,*,#3346,.F.);
#4497=ORIENTED_EDGE('',*,*,#3347,.F.);
#4498=ORIENTED_EDGE('',*,*,#3348,.F.);
#4499=ORIENTED_EDGE('',*,*,#3347,.T.);
#4500=ORIENTED_EDGE('',*,*,#3349,.F.);
#4501=ORIENTED_EDGE('',*,*,#3350,.F.);
#4502=ORIENTED_EDGE('',*,*,#3351,.F.);
#4503=ORIENTED_EDGE('',*,*,#3350,.T.);
#4504=ORIENTED_EDGE('',*,*,#3352,.F.);
#4505=ORIENTED_EDGE('',*,*,#3353,.F.);
#4506=ORIENTED_EDGE('',*,*,#3354,.F.);
#4507=ORIENTED_EDGE('',*,*,#3353,.T.);
#4508=ORIENTED_EDGE('',*,*,#3355,.F.);
#4509=ORIENTED_EDGE('',*,*,#3356,.F.);
#4510=ORIENTED_EDGE('',*,*,#3357,.F.);
#4511=ORIENTED_EDGE('',*,*,#3356,.T.);
#4512=ORIENTED_EDGE('',*,*,#3358,.F.);
#4513=ORIENTED_EDGE('',*,*,#3359,.F.);
#4514=ORIENTED_EDGE('',*,*,#3360,.F.);
#4515=ORIENTED_EDGE('',*,*,#3359,.T.);
#4516=ORIENTED_EDGE('',*,*,#3361,.F.);
#4517=ORIENTED_EDGE('',*,*,#3362,.F.);
#4518=ORIENTED_EDGE('',*,*,#3363,.F.);
#4519=ORIENTED_EDGE('',*,*,#3362,.T.);
#4520=ORIENTED_EDGE('',*,*,#3364,.F.);
#4521=ORIENTED_EDGE('',*,*,#3365,.F.);
#4522=ORIENTED_EDGE('',*,*,#3366,.F.);
#4523=ORIENTED_EDGE('',*,*,#3365,.T.);
#4524=ORIENTED_EDGE('',*,*,#3367,.F.);
#4525=ORIENTED_EDGE('',*,*,#3368,.F.);
#4526=ORIENTED_EDGE('',*,*,#3369,.F.);
#4527=ORIENTED_EDGE('',*,*,#3368,.T.);
#4528=ORIENTED_EDGE('',*,*,#3370,.F.);
#4529=ORIENTED_EDGE('',*,*,#3371,.F.);
#4530=ORIENTED_EDGE('',*,*,#3372,.F.);
#4531=ORIENTED_EDGE('',*,*,#3371,.T.);
#4532=ORIENTED_EDGE('',*,*,#3373,.F.);
#4533=ORIENTED_EDGE('',*,*,#3374,.F.);
#4534=ORIENTED_EDGE('',*,*,#3375,.F.);
#4535=ORIENTED_EDGE('',*,*,#3374,.T.);
#4536=ORIENTED_EDGE('',*,*,#3376,.F.);
#4537=ORIENTED_EDGE('',*,*,#3377,.F.);
#4538=ORIENTED_EDGE('',*,*,#3378,.F.);
#4539=ORIENTED_EDGE('',*,*,#3377,.T.);
#4540=ORIENTED_EDGE('',*,*,#3379,.F.);
#4541=ORIENTED_EDGE('',*,*,#3237,.F.);
#4542=ORIENTED_EDGE('',*,*,#3379,.T.);
#4543=ORIENTED_EDGE('',*,*,#3376,.T.);
#4544=ORIENTED_EDGE('',*,*,#3373,.T.);
#4545=ORIENTED_EDGE('',*,*,#3370,.T.);
#4546=ORIENTED_EDGE('',*,*,#3367,.T.);
#4547=ORIENTED_EDGE('',*,*,#3364,.T.);
#4548=ORIENTED_EDGE('',*,*,#3361,.T.);
#4549=ORIENTED_EDGE('',*,*,#3358,.T.);
#4550=ORIENTED_EDGE('',*,*,#3355,.T.);
#4551=ORIENTED_EDGE('',*,*,#3352,.T.);
#4552=ORIENTED_EDGE('',*,*,#3349,.T.);
#4553=ORIENTED_EDGE('',*,*,#3346,.T.);
#4554=ORIENTED_EDGE('',*,*,#3343,.T.);
#4555=ORIENTED_EDGE('',*,*,#3340,.T.);
#4556=ORIENTED_EDGE('',*,*,#3337,.T.);
#4557=ORIENTED_EDGE('',*,*,#3334,.T.);
#4558=ORIENTED_EDGE('',*,*,#3331,.T.);
#4559=ORIENTED_EDGE('',*,*,#3328,.T.);
#4560=ORIENTED_EDGE('',*,*,#3325,.T.);
#4561=ORIENTED_EDGE('',*,*,#3322,.T.);
#4562=ORIENTED_EDGE('',*,*,#3319,.T.);
#4563=ORIENTED_EDGE('',*,*,#3316,.T.);
#4564=ORIENTED_EDGE('',*,*,#3313,.T.);
#4565=ORIENTED_EDGE('',*,*,#3310,.T.);
#4566=ORIENTED_EDGE('',*,*,#3307,.T.);
#4567=ORIENTED_EDGE('',*,*,#3304,.T.);
#4568=ORIENTED_EDGE('',*,*,#3301,.T.);
#4569=ORIENTED_EDGE('',*,*,#3298,.T.);
#4570=ORIENTED_EDGE('',*,*,#3295,.T.);
#4571=ORIENTED_EDGE('',*,*,#3292,.T.);
#4572=ORIENTED_EDGE('',*,*,#3289,.T.);
#4573=ORIENTED_EDGE('',*,*,#3286,.T.);
#4574=ORIENTED_EDGE('',*,*,#3283,.T.);
#4575=ORIENTED_EDGE('',*,*,#3280,.T.);
#4576=ORIENTED_EDGE('',*,*,#3277,.T.);
#4577=ORIENTED_EDGE('',*,*,#3274,.T.);
#4578=ORIENTED_EDGE('',*,*,#3271,.T.);
#4579=ORIENTED_EDGE('',*,*,#3268,.T.);
#4580=ORIENTED_EDGE('',*,*,#3265,.T.);
#4581=ORIENTED_EDGE('',*,*,#3262,.T.);
#4582=ORIENTED_EDGE('',*,*,#3259,.T.);
#4583=ORIENTED_EDGE('',*,*,#3256,.T.);
#4584=ORIENTED_EDGE('',*,*,#3253,.T.);
#4585=ORIENTED_EDGE('',*,*,#3250,.T.);
#4586=ORIENTED_EDGE('',*,*,#3247,.T.);
#4587=ORIENTED_EDGE('',*,*,#3244,.T.);
#4588=ORIENTED_EDGE('',*,*,#3241,.T.);
#4589=ORIENTED_EDGE('',*,*,#3238,.T.);
#4590=ORIENTED_EDGE('',*,*,#3232,.T.);
#4591=ORIENTED_EDGE('',*,*,#3378,.T.);
#4592=ORIENTED_EDGE('',*,*,#3236,.T.);
#4593=ORIENTED_EDGE('',*,*,#3240,.T.);
#4594=ORIENTED_EDGE('',*,*,#3243,.T.);
#4595=ORIENTED_EDGE('',*,*,#3246,.T.);
#4596=ORIENTED_EDGE('',*,*,#3249,.T.);
#4597=ORIENTED_EDGE('',*,*,#3252,.T.);
#4598=ORIENTED_EDGE('',*,*,#3255,.T.);
#4599=ORIENTED_EDGE('',*,*,#3258,.T.);
#4600=ORIENTED_EDGE('',*,*,#3261,.T.);
#4601=ORIENTED_EDGE('',*,*,#3264,.T.);
#4602=ORIENTED_EDGE('',*,*,#3267,.T.);
#4603=ORIENTED_EDGE('',*,*,#3270,.T.);
#4604=ORIENTED_EDGE('',*,*,#3273,.T.);
#4605=ORIENTED_EDGE('',*,*,#3276,.T.);
#4606=ORIENTED_EDGE('',*,*,#3279,.T.);
#4607=ORIENTED_EDGE('',*,*,#3282,.T.);
#4608=ORIENTED_EDGE('',*,*,#3285,.T.);
#4609=ORIENTED_EDGE('',*,*,#3288,.T.);
#4610=ORIENTED_EDGE('',*,*,#3291,.T.);
#4611=ORIENTED_EDGE('',*,*,#3294,.T.);
#4612=ORIENTED_EDGE('',*,*,#3297,.T.);
#4613=ORIENTED_EDGE('',*,*,#3300,.T.);
#4614=ORIENTED_EDGE('',*,*,#3303,.T.);
#4615=ORIENTED_EDGE('',*,*,#3306,.T.);
#4616=ORIENTED_EDGE('',*,*,#3309,.T.);
#4617=ORIENTED_EDGE('',*,*,#3312,.T.);
#4618=ORIENTED_EDGE('',*,*,#3315,.T.);
#4619=ORIENTED_EDGE('',*,*,#3318,.T.);
#4620=ORIENTED_EDGE('',*,*,#3321,.T.);
#4621=ORIENTED_EDGE('',*,*,#3324,.T.);
#4622=ORIENTED_EDGE('',*,*,#3327,.T.);
#4623=ORIENTED_EDGE('',*,*,#3330,.T.);
#4624=ORIENTED_EDGE('',*,*,#3333,.T.);
#4625=ORIENTED_EDGE('',*,*,#3336,.T.);
#4626=ORIENTED_EDGE('',*,*,#3339,.T.);
#4627=ORIENTED_EDGE('',*,*,#3342,.T.);
#4628=ORIENTED_EDGE('',*,*,#3345,.T.);
#4629=ORIENTED_EDGE('',*,*,#3348,.T.);
#4630=ORIENTED_EDGE('',*,*,#3351,.T.);
#4631=ORIENTED_EDGE('',*,*,#3354,.T.);
#4632=ORIENTED_EDGE('',*,*,#3357,.T.);
#4633=ORIENTED_EDGE('',*,*,#3360,.T.);
#4634=ORIENTED_EDGE('',*,*,#3363,.T.);
#4635=ORIENTED_EDGE('',*,*,#3366,.T.);
#4636=ORIENTED_EDGE('',*,*,#3369,.T.);
#4637=ORIENTED_EDGE('',*,*,#3372,.T.);
#4638=ORIENTED_EDGE('',*,*,#3375,.T.);
#4639=ORIENTED_EDGE('',*,*,#3234,.T.);
#4841=CYLINDRICAL_SURFACE('',#5950,0.21);
#4842=CYLINDRICAL_SURFACE('',#5954,1.6);
#4843=CYLINDRICAL_SURFACE('',#5959,1.005);
#5070=ADVANCED_FACE('',(#844),#549,.T.);
#5071=ADVANCED_FACE('',(#845),#4841,.F.);
#5072=ADVANCED_FACE('',(#846),#550,.T.);
#5073=ADVANCED_FACE('',(#847,#429),#4842,.T.);
#5074=ADVANCED_FACE('',(#848,#430),#551,.T.);
#5075=ADVANCED_FACE('',(#849,#431),#4843,.F.);
#5076=ADVANCED_FACE('',(#850),#552,.T.);
#5077=ADVANCED_FACE('',(#851),#553,.T.);
#5078=ADVANCED_FACE('',(#852),#554,.T.);
#5079=ADVANCED_FACE('',(#853),#555,.T.);
#5080=ADVANCED_FACE('',(#854),#556,.T.);
#5081=ADVANCED_FACE('',(#855),#557,.T.);
#5082=ADVANCED_FACE('',(#856),#558,.T.);
#5083=ADVANCED_FACE('',(#857),#559,.T.);
#5084=ADVANCED_FACE('',(#858),#560,.T.);
#5085=ADVANCED_FACE('',(#859),#561,.T.);
#5086=ADVANCED_FACE('',(#860),#562,.T.);
#5087=ADVANCED_FACE('',(#861),#563,.T.);
#5088=ADVANCED_FACE('',(#862),#564,.T.);
#5089=ADVANCED_FACE('',(#863),#565,.T.);
#5090=ADVANCED_FACE('',(#864),#566,.T.);
#5091=ADVANCED_FACE('',(#865),#567,.T.);
#5092=ADVANCED_FACE('',(#866),#568,.T.);
#5093=ADVANCED_FACE('',(#867),#569,.T.);
#5094=ADVANCED_FACE('',(#868),#570,.T.);
#5095=ADVANCED_FACE('',(#869),#571,.T.);
#5096=ADVANCED_FACE('',(#870),#572,.T.);
#5097=ADVANCED_FACE('',(#871),#573,.T.);
#5098=ADVANCED_FACE('',(#872),#574,.T.);
#5099=ADVANCED_FACE('',(#873),#575,.T.);
#5100=ADVANCED_FACE('',(#874),#576,.T.);
#5101=ADVANCED_FACE('',(#875),#577,.T.);
#5102=ADVANCED_FACE('',(#876),#578,.T.);
#5103=ADVANCED_FACE('',(#877),#579,.T.);
#5104=ADVANCED_FACE('',(#878),#580,.T.);
#5105=ADVANCED_FACE('',(#879),#581,.T.);
#5106=ADVANCED_FACE('',(#880),#582,.T.);
#5107=ADVANCED_FACE('',(#881),#583,.T.);
#5108=ADVANCED_FACE('',(#882),#584,.T.);
#5109=ADVANCED_FACE('',(#883),#585,.T.);
#5110=ADVANCED_FACE('',(#884),#586,.T.);
#5111=ADVANCED_FACE('',(#885),#587,.T.);
#5112=ADVANCED_FACE('',(#886),#588,.T.);
#5113=ADVANCED_FACE('',(#887),#589,.T.);
#5114=ADVANCED_FACE('',(#888),#590,.T.);
#5115=ADVANCED_FACE('',(#889),#591,.T.);
#5116=ADVANCED_FACE('',(#890),#592,.T.);
#5117=ADVANCED_FACE('',(#891),#593,.T.);
#5118=ADVANCED_FACE('',(#892),#594,.T.);
#5119=ADVANCED_FACE('',(#893),#595,.T.);
#5120=ADVANCED_FACE('',(#894),#596,.T.);
#5121=ADVANCED_FACE('',(#895),#597,.T.);
#5122=ADVANCED_FACE('',(#896),#598,.T.);
#5123=ADVANCED_FACE('',(#897),#599,.T.);
#5124=ADVANCED_FACE('',(#898,#432),#600,.T.);
#5125=ADVANCED_FACE('',(#899,#433),#601,.F.);
#5185=CLOSED_SHELL('',(#5070,#5071,#5072,#5073,#5074,#5075,#5076,#5077,
#5078,#5079,#5080,#5081,#5082,#5083,#5084,#5085,#5086,#5087,#5088,#5089,
#5090,#5091,#5092,#5093,#5094,#5095,#5096,#5097,#5098,#5099,#5100,#5101,
#5102,#5103,#5104,#5105,#5106,#5107,#5108,#5109,#5110,#5111,#5112,#5113,
#5114,#5115,#5116,#5117,#5118,#5119,#5120,#5121,#5122,#5123,#5124,#5125));
#5947=AXIS2_PLACEMENT_3D('',#10673,#7240,#7241);
#5948=AXIS2_PLACEMENT_3D('',#10674,#7242,#7243);
#5949=AXIS2_PLACEMENT_3D('',#10678,#7245,#7246);
#5950=AXIS2_PLACEMENT_3D('',#10679,#7247,#7248);
#5951=AXIS2_PLACEMENT_3D('',#10696,#7249,#7250);
#5952=AXIS2_PLACEMENT_3D('',#10737,#7252,#7253);
#5953=AXIS2_PLACEMENT_3D('',#10752,#7254,#7255);
#5954=AXIS2_PLACEMENT_3D('',#10754,#7257,#7258);
#5955=AXIS2_PLACEMENT_3D('',#10756,#7259,#7260);
#5956=AXIS2_PLACEMENT_3D('',#10759,#7262,#7263);
#5957=AXIS2_PLACEMENT_3D('',#10760,#7264,#7265);
#5958=AXIS2_PLACEMENT_3D('',#10762,#7266,#7267);
#5959=AXIS2_PLACEMENT_3D('',#10763,#7268,#7269);
#5960=AXIS2_PLACEMENT_3D('',#10765,#7270,#7271);
#5961=AXIS2_PLACEMENT_3D('',#10767,#7273,#7274);
#5962=AXIS2_PLACEMENT_3D('',#10776,#7279,#7280);
#5963=AXIS2_PLACEMENT_3D('',#10782,#7284,#7285);
#5964=AXIS2_PLACEMENT_3D('',#10788,#7289,#7290);
#5965=AXIS2_PLACEMENT_3D('',#10794,#7294,#7295);
#5966=AXIS2_PLACEMENT_3D('',#10800,#7299,#7300);
#5967=AXIS2_PLACEMENT_3D('',#10806,#7304,#7305);
#5968=AXIS2_PLACEMENT_3D('',#10812,#7309,#7310);
#5969=AXIS2_PLACEMENT_3D('',#10818,#7314,#7315);
#5970=AXIS2_PLACEMENT_3D('',#10824,#7319,#7320);
#5971=AXIS2_PLACEMENT_3D('',#10830,#7324,#7325);
#5972=AXIS2_PLACEMENT_3D('',#10836,#7329,#7330);
#5973=AXIS2_PLACEMENT_3D('',#10842,#7334,#7335);
#5974=AXIS2_PLACEMENT_3D('',#10848,#7339,#7340);
#5975=AXIS2_PLACEMENT_3D('',#10854,#7344,#7345);
#5976=AXIS2_PLACEMENT_3D('',#10860,#7349,#7350);
#5977=AXIS2_PLACEMENT_3D('',#10866,#7354,#7355);
#5978=AXIS2_PLACEMENT_3D('',#10872,#7359,#7360);
#5979=AXIS2_PLACEMENT_3D('',#10878,#7364,#7365);
#5980=AXIS2_PLACEMENT_3D('',#10884,#7369,#7370);
#5981=AXIS2_PLACEMENT_3D('',#10890,#7374,#7375);
#5982=AXIS2_PLACEMENT_3D('',#10896,#7379,#7380);
#5983=AXIS2_PLACEMENT_3D('',#10902,#7384,#7385);
#5984=AXIS2_PLACEMENT_3D('',#10908,#7389,#7390);
#5985=AXIS2_PLACEMENT_3D('',#10914,#7394,#7395);
#5986=AXIS2_PLACEMENT_3D('',#10920,#7399,#7400);
#5987=AXIS2_PLACEMENT_3D('',#10926,#7404,#7405);
#5988=AXIS2_PLACEMENT_3D('',#10932,#7409,#7410);
#5989=AXIS2_PLACEMENT_3D('',#10938,#7414,#7415);
#5990=AXIS2_PLACEMENT_3D('',#10944,#7419,#7420);
#5991=AXIS2_PLACEMENT_3D('',#10950,#7424,#7425);
#5992=AXIS2_PLACEMENT_3D('',#10956,#7429,#7430);
#5993=AXIS2_PLACEMENT_3D('',#10962,#7434,#7435);
#5994=AXIS2_PLACEMENT_3D('',#10968,#7439,#7440);
#5995=AXIS2_PLACEMENT_3D('',#10974,#7444,#7445);
#5996=AXIS2_PLACEMENT_3D('',#10980,#7449,#7450);
#5997=AXIS2_PLACEMENT_3D('',#10986,#7454,#7455);
#5998=AXIS2_PLACEMENT_3D('',#10992,#7459,#7460);
#5999=AXIS2_PLACEMENT_3D('',#10998,#7464,#7465);
#6000=AXIS2_PLACEMENT_3D('',#11004,#7469,#7470);
#6001=AXIS2_PLACEMENT_3D('',#11010,#7474,#7475);
#6002=AXIS2_PLACEMENT_3D('',#11016,#7479,#7480);
#6003=AXIS2_PLACEMENT_3D('',#11022,#7484,#7485);
#6004=AXIS2_PLACEMENT_3D('',#11028,#7489,#7490);
#6005=AXIS2_PLACEMENT_3D('',#11034,#7494,#7495);
#6006=AXIS2_PLACEMENT_3D('',#11040,#7499,#7500);
#6007=AXIS2_PLACEMENT_3D('',#11046,#7504,#7505);
#6008=AXIS2_PLACEMENT_3D('',#11052,#7509,#7510);
#6009=AXIS2_PLACEMENT_3D('',#11055,#7513,#7514);
#6010=AXIS2_PLACEMENT_3D('',#11056,#7515,#7516);
#7240=DIRECTION('axis',(0.,0.,1.));
#7241=DIRECTION('refdir',(1.,0.,0.));
#7242=DIRECTION('center_axis',(0.,0.,1.));
#7243=DIRECTION('ref_axis',(1.,0.,0.));
#7244=DIRECTION('',(0.,1.,0.));
#7245=DIRECTION('center_axis',(0.,0.,1.));
#7246=DIRECTION('ref_axis',(1.,0.,0.));
#7247=DIRECTION('center_axis',(0.,0.,1.));
#7248=DIRECTION('ref_axis',(1.,0.,0.));
#7249=DIRECTION('center_axis',(0.,0.,1.));
#7250=DIRECTION('ref_axis',(1.,0.,0.));
#7251=DIRECTION('',(0.,0.,1.));
#7252=DIRECTION('center_axis',(0.,0.,1.));
#7253=DIRECTION('ref_axis',(1.,0.,0.));
#7254=DIRECTION('center_axis',(0.,0.,1.));
#7255=DIRECTION('ref_axis',(1.,0.,0.));
#7256=DIRECTION('',(0.,-1.,0.));
#7257=DIRECTION('center_axis',(0.,1.,0.));
#7258=DIRECTION('ref_axis',(1.,0.,0.));
#7259=DIRECTION('center_axis',(0.,1.,0.));
#7260=DIRECTION('ref_axis',(1.,0.,0.));
#7261=DIRECTION('',(0.,-1.,0.));
#7262=DIRECTION('center_axis',(0.,-1.,0.));
#7263=DIRECTION('ref_axis',(1.,0.,0.));
#7264=DIRECTION('center_axis',(0.,1.,0.));
#7265=DIRECTION('ref_axis',(1.,0.,0.));
#7266=DIRECTION('center_axis',(0.,-1.,0.));
#7267=DIRECTION('ref_axis',(1.,0.,0.));
#7268=DIRECTION('center_axis',(0.,1.,0.));
#7269=DIRECTION('ref_axis',(1.,0.,0.));
#7270=DIRECTION('center_axis',(0.,1.,0.));
#7271=DIRECTION('ref_axis',(1.,0.,0.));
#7272=DIRECTION('',(0.,1.,0.));
#7273=DIRECTION('center_axis',(0.015706233006771,0.,0.999876649514697));
#7274=DIRECTION('ref_axis',(0.999876649514697,0.,-0.015706233006771));
#7275=DIRECTION('',(-0.999876649514697,0.,0.015706233006771));
#7276=DIRECTION('',(0.,1.,0.));
#7277=DIRECTION('',(0.999876649514697,0.,-0.015706233006771));
#7278=DIRECTION('',(0.,1.,0.));
#7279=DIRECTION('center_axis',(0.957469564385932,0.,-0.288534284400681));
#7280=DIRECTION('ref_axis',(-0.288534284400681,0.,-0.957469564385932));
#7281=DIRECTION('',(0.288534284400681,0.,0.957469564385932));
#7282=DIRECTION('',(-0.288534284400681,0.,-0.957469564385932));
#7283=DIRECTION('',(0.,1.,0.));
#7284=DIRECTION('center_axis',(-0.243616063552747,0.,0.9698717510986));
#7285=DIRECTION('ref_axis',(0.9698717510986,0.,0.243616063552747));
#7286=DIRECTION('',(-0.9698717510986,0.,-0.243616063552747));
#7287=DIRECTION('',(0.9698717510986,0.,0.243616063552747));
#7288=DIRECTION('',(0.,1.,0.));
#7289=DIRECTION('center_axis',(0.999522748094039,0.,-0.0308913587033594));
#7290=DIRECTION('ref_axis',(-0.0308913587033594,0.,-0.999522748094039));
#7291=DIRECTION('',(0.0308913587033594,0.,0.999522748094039));
#7292=DIRECTION('',(-0.0308913587033594,0.,-0.999522748094039));
#7293=DIRECTION('',(0.,1.,0.));
#7294=DIRECTION('center_axis',(-0.486336327975727,0.,0.873771695633983));
#7295=DIRECTION('ref_axis',(0.873771695633983,0.,0.486336327975727));
#7296=DIRECTION('',(-0.873771695633983,0.,-0.486336327975727));
#7297=DIRECTION('',(0.873771695633983,0.,0.486336327975727));
#7298=DIRECTION('',(0.,1.,0.));
#7299=DIRECTION('center_axis',(0.973460108308978,0.,0.228856762039213));
#7300=DIRECTION('ref_axis',(0.228856762039213,0.,-0.973460108308978));
#7301=DIRECTION('',(-0.228856762039213,0.,0.973460108308978));
#7302=DIRECTION('',(0.228856762039213,0.,-0.973460108308978));
#7303=DIRECTION('',(0.,1.,0.));
#7304=DIRECTION('center_axis',(-0.695913575355945,0.,0.71812554308791));
#7305=DIRECTION('ref_axis',(0.71812554308791,0.,0.695913575355945));
#7306=DIRECTION('',(-0.71812554308791,0.,-0.695913575355945));
#7307=DIRECTION('',(0.71812554308791,0.,0.695913575355945));
#7308=DIRECTION('',(0.,1.,0.));
#7309=DIRECTION('center_axis',(0.881057770861552,0.,0.473008672652493));
#7310=DIRECTION('ref_axis',(0.473008672652493,0.,-0.881057770861552));
#7311=DIRECTION('',(-0.473008672652493,0.,0.881057770861552));
#7312=DIRECTION('',(0.473008672652493,0.,-0.881057770861552));
#7313=DIRECTION('',(0.,1.,0.));
#7314=DIRECTION('center_axis',(-0.858065462627213,0.,0.513540321538968));
#7315=DIRECTION('ref_axis',(0.513540321538968,0.,0.858065462627213));
#7316=DIRECTION('',(-0.513540321538968,0.,-0.858065462627213));
#7317=DIRECTION('',(0.513540321538968,0.,0.858065462627213));
#7318=DIRECTION('',(0.,1.,0.));
#7319=DIRECTION('center_axis',(0.728612802346719,0.,0.684925823908298));
#7320=DIRECTION('ref_axis',(0.684925823908298,0.,-0.728612802346719));
#7321=DIRECTION('',(-0.684925823908298,0.,0.728612802346719));
#7322=DIRECTION('',(0.684925823908298,0.,-0.728612802346719));
#7323=DIRECTION('',(0.,1.,0.));
#7324=DIRECTION('center_axis',(-0.96174160664066,0.,0.273958175742654));
#7325=DIRECTION('ref_axis',(0.273958175742654,0.,0.96174160664066));
#7326=DIRECTION('',(-0.273958175742654,0.,-0.96174160664066));
#7327=DIRECTION('',(0.273958175742654,0.,0.96174160664066));
#7328=DIRECTION('',(0.,1.,0.));
#7329=DIRECTION('center_axis',(0.526514075441545,0.,0.850166412158193));
#7330=DIRECTION('ref_axis',(0.850166412158193,0.,-0.526514075441545));
#7331=DIRECTION('',(-0.850166412158193,0.,0.526514075441545));
#7332=DIRECTION('',(0.850166412158193,0.,-0.526514075441545));
#7333=DIRECTION('',(0.,1.,0.));
#7334=DIRECTION('center_axis',(-0.999876649514698,0.,0.0157062330067685));
#7335=DIRECTION('ref_axis',(0.0157062330067685,0.,0.999876649514698));
#7336=DIRECTION('',(-0.0157062330067685,0.,-0.999876649514698));
#7337=DIRECTION('',(0.0157062330067685,0.,0.999876649514698));
#7338=DIRECTION('',(0.,1.,0.));
#7339=DIRECTION('center_axis',(0.288534284400681,0.,0.957469564385932));
#7340=DIRECTION('ref_axis',(0.957469564385932,0.,-0.288534284400681));
#7341=DIRECTION('',(-0.957469564385932,0.,0.288534284400681));
#7342=DIRECTION('',(0.957469564385932,0.,-0.288534284400681));
#7343=DIRECTION('',(0.,1.,0.));
#7344=DIRECTION('center_axis',(-0.969871751098599,0.,-0.243616063552749));
#7345=DIRECTION('ref_axis',(-0.243616063552749,0.,0.969871751098599));
#7346=DIRECTION('',(0.243616063552749,0.,-0.969871751098599));
#7347=DIRECTION('',(-0.243616063552749,0.,0.969871751098599));
#7348=DIRECTION('',(0.,1.,0.));
#7349=DIRECTION('center_axis',(0.0308913587033598,0.,0.999522748094039));
#7350=DIRECTION('ref_axis',(0.999522748094039,0.,-0.0308913587033598));
#7351=DIRECTION('',(-0.999522748094039,0.,0.0308913587033598));
#7352=DIRECTION('',(0.999522748094039,0.,-0.0308913587033598));
#7353=DIRECTION('',(0.,1.,0.));
#7354=DIRECTION('center_axis',(-0.873771695633983,0.,-0.486336327975728));
#7355=DIRECTION('ref_axis',(-0.486336327975728,0.,0.873771695633983));
#7356=DIRECTION('',(0.486336327975728,0.,-0.873771695633983));
#7357=DIRECTION('',(-0.486336327975728,0.,0.873771695633983));
#7358=DIRECTION('',(0.,1.,0.));
#7359=DIRECTION('center_axis',(-0.228856762039212,0.,0.973460108308978));
#7360=DIRECTION('ref_axis',(0.973460108308978,0.,0.228856762039212));
#7361=DIRECTION('',(-0.973460108308978,0.,-0.228856762039212));
#7362=DIRECTION('',(0.973460108308978,0.,0.228856762039212));
#7363=DIRECTION('',(0.,1.,0.));
#7364=DIRECTION('center_axis',(-0.718125543087911,0.,-0.695913575355944));
#7365=DIRECTION('ref_axis',(-0.695913575355944,0.,0.718125543087911));
#7366=DIRECTION('',(0.695913575355944,0.,-0.718125543087911));
#7367=DIRECTION('',(-0.695913575355944,0.,0.718125543087911));
#7368=DIRECTION('',(0.,1.,0.));
#7369=DIRECTION('center_axis',(-0.473008672652494,0.,0.881057770861551));
#7370=DIRECTION('ref_axis',(0.881057770861551,0.,0.473008672652494));
#7371=DIRECTION('',(-0.881057770861551,0.,-0.473008672652494));
#7372=DIRECTION('',(0.881057770861551,0.,0.473008672652494));
#7373=DIRECTION('',(0.,1.,0.));
#7374=DIRECTION('center_axis',(-0.513540321538967,0.,-0.858065462627214));
#7375=DIRECTION('ref_axis',(-0.858065462627214,0.,0.513540321538967));
#7376=DIRECTION('',(0.858065462627214,0.,-0.513540321538967));
#7377=DIRECTION('',(-0.858065462627214,0.,0.513540321538967));
#7378=DIRECTION('',(0.,1.,0.));
#7379=DIRECTION('center_axis',(-0.684925823908296,0.,0.728612802346721));
#7380=DIRECTION('ref_axis',(0.728612802346721,0.,0.684925823908296));
#7381=DIRECTION('',(-0.728612802346721,0.,-0.684925823908296));
#7382=DIRECTION('',(0.728612802346721,0.,0.684925823908296));
#7383=DIRECTION('',(0.,1.,0.));
#7384=DIRECTION('center_axis',(-0.273958175742656,0.,-0.961741606640659));
#7385=DIRECTION('ref_axis',(-0.961741606640659,0.,0.273958175742656));
#7386=DIRECTION('',(0.961741606640659,0.,-0.273958175742656));
#7387=DIRECTION('',(-0.961741606640659,0.,0.273958175742656));
#7388=DIRECTION('',(0.,1.,0.));
#7389=DIRECTION('center_axis',(-0.850166412158193,0.,0.526514075441546));
#7390=DIRECTION('ref_axis',(0.526514075441546,0.,0.850166412158193));
#7391=DIRECTION('',(-0.526514075441546,0.,-0.850166412158193));
#7392=DIRECTION('',(0.526514075441546,0.,0.850166412158193));
#7393=DIRECTION('',(0.,1.,0.));
#7394=DIRECTION('center_axis',(-0.0157062330067692,0.,-0.999876649514697));
#7395=DIRECTION('ref_axis',(-0.999876649514697,0.,0.0157062330067692));
#7396=DIRECTION('',(0.999876649514697,0.,-0.0157062330067692));
#7397=DIRECTION('',(-0.999876649514697,0.,0.0157062330067692));
#7398=DIRECTION('',(0.,1.,0.));
#7399=DIRECTION('center_axis',(-0.957469564385932,0.,0.288534284400681));
#7400=DIRECTION('ref_axis',(0.288534284400681,0.,0.957469564385932));
#7401=DIRECTION('',(-0.288534284400681,0.,-0.957469564385932));
#7402=DIRECTION('',(0.288534284400681,0.,0.957469564385932));
#7403=DIRECTION('',(0.,1.,0.));
#7404=DIRECTION('center_axis',(0.24361606355275,0.,-0.969871751098599));
#7405=DIRECTION('ref_axis',(-0.969871751098599,0.,-0.24361606355275));
#7406=DIRECTION('',(0.969871751098599,0.,0.24361606355275));
#7407=DIRECTION('',(-0.969871751098599,0.,-0.24361606355275));
#7408=DIRECTION('',(0.,1.,0.));
#7409=DIRECTION('center_axis',(-0.999522748094039,0.,0.0308913587033594));
#7410=DIRECTION('ref_axis',(0.0308913587033594,0.,0.999522748094039));
#7411=DIRECTION('',(-0.0308913587033594,0.,-0.999522748094039));
#7412=DIRECTION('',(0.0308913587033594,0.,0.999522748094039));
#7413=DIRECTION('',(0.,1.,0.));
#7414=DIRECTION('center_axis',(0.486336327975727,0.,-0.873771695633983));
#7415=DIRECTION('ref_axis',(-0.873771695633983,0.,-0.486336327975727));
#7416=DIRECTION('',(0.873771695633983,0.,0.486336327975727));
#7417=DIRECTION('',(-0.873771695633983,0.,-0.486336327975727));
#7418=DIRECTION('',(0.,1.,0.));
#7419=DIRECTION('center_axis',(-0.973460108308978,0.,-0.228856762039212));
#7420=DIRECTION('ref_axis',(-0.228856762039212,0.,0.973460108308978));
#7421=DIRECTION('',(0.228856762039212,0.,-0.973460108308978));
#7422=DIRECTION('',(-0.228856762039212,0.,0.973460108308978));
#7423=DIRECTION('',(0.,1.,0.));
#7424=DIRECTION('center_axis',(0.695913575355945,0.,-0.718125543087909));
#7425=DIRECTION('ref_axis',(-0.718125543087909,0.,-0.695913575355945));
#7426=DIRECTION('',(0.718125543087909,0.,0.695913575355945));
#7427=DIRECTION('',(-0.718125543087909,0.,-0.695913575355945));
#7428=DIRECTION('',(0.,1.,0.));
#7429=DIRECTION('center_axis',(-0.881057770861552,0.,-0.473008672652493));
#7430=DIRECTION('ref_axis',(-0.473008672652493,0.,0.881057770861552));
#7431=DIRECTION('',(0.473008672652493,0.,-0.881057770861552));
#7432=DIRECTION('',(-0.473008672652493,0.,0.881057770861552));
#7433=DIRECTION('',(0.,1.,0.));
#7434=DIRECTION('center_axis',(0.858065462627214,0.,-0.513540321538968));
#7435=DIRECTION('ref_axis',(-0.513540321538968,0.,-0.858065462627214));
#7436=DIRECTION('',(0.513540321538968,0.,0.858065462627214));
#7437=DIRECTION('',(-0.513540321538968,0.,-0.858065462627214));
#7438=DIRECTION('',(0.,1.,0.));
#7439=DIRECTION('center_axis',(-0.728612802346719,0.,-0.684925823908298));
#7440=DIRECTION('ref_axis',(-0.684925823908298,0.,0.728612802346719));
#7441=DIRECTION('',(0.684925823908298,0.,-0.728612802346719));
#7442=DIRECTION('',(-0.684925823908298,0.,0.728612802346719));
#7443=DIRECTION('',(0.,1.,0.));
#7444=DIRECTION('center_axis',(0.96174160664066,0.,-0.273958175742653));
#7445=DIRECTION('ref_axis',(-0.273958175742653,0.,-0.96174160664066));
#7446=DIRECTION('',(0.273958175742653,0.,0.96174160664066));
#7447=DIRECTION('',(-0.273958175742653,0.,-0.96174160664066));
#7448=DIRECTION('',(0.,1.,0.));
#7449=DIRECTION('center_axis',(-0.526514075441546,0.,-0.850166412158193));
#7450=DIRECTION('ref_axis',(-0.850166412158193,0.,0.526514075441546));
#7451=DIRECTION('',(0.850166412158193,0.,-0.526514075441546));
#7452=DIRECTION('',(-0.850166412158193,0.,0.526514075441546));
#7453=DIRECTION('',(0.,1.,0.));
#7454=DIRECTION('center_axis',(0.999876649514698,0.,-0.0157062330067686));
#7455=DIRECTION('ref_axis',(-0.0157062330067686,0.,-0.999876649514698));
#7456=DIRECTION('',(0.0157062330067686,0.,0.999876649514698));
#7457=DIRECTION('',(-0.0157062330067686,0.,-0.999876649514698));
#7458=DIRECTION('',(0.,1.,0.));
#7459=DIRECTION('center_axis',(-0.288534284400682,0.,-0.957469564385932));
#7460=DIRECTION('ref_axis',(-0.957469564385932,0.,0.288534284400682));
#7461=DIRECTION('',(0.957469564385932,0.,-0.288534284400682));
#7462=DIRECTION('',(-0.957469564385932,0.,0.288534284400682));
#7463=DIRECTION('',(0.,1.,0.));
#7464=DIRECTION('center_axis',(0.969871751098599,0.,0.24361606355275));
#7465=DIRECTION('ref_axis',(0.24361606355275,0.,-0.969871751098599));
#7466=DIRECTION('',(-0.24361606355275,0.,0.969871751098599));
#7467=DIRECTION('',(0.24361606355275,0.,-0.969871751098599));
#7468=DIRECTION('',(0.,1.,0.));
#7469=DIRECTION('center_axis',(-0.0308913587033594,0.,-0.999522748094039));
#7470=DIRECTION('ref_axis',(-0.999522748094039,0.,0.0308913587033594));
#7471=DIRECTION('',(0.999522748094039,0.,-0.0308913587033594));
#7472=DIRECTION('',(-0.999522748094039,0.,0.0308913587033594));
#7473=DIRECTION('',(0.,1.,0.));
#7474=DIRECTION('center_axis',(0.873771695633986,0.,0.486336327975723));
#7475=DIRECTION('ref_axis',(0.486336327975723,0.,-0.873771695633986));
#7476=DIRECTION('',(-0.486336327975723,0.,0.873771695633986));
#7477=DIRECTION('',(0.486336327975723,0.,-0.873771695633986));
#7478=DIRECTION('',(0.,1.,0.));
#7479=DIRECTION('center_axis',(0.228856762039213,0.,-0.973460108308978));
#7480=DIRECTION('ref_axis',(-0.973460108308978,0.,-0.228856762039213));
#7481=DIRECTION('',(0.973460108308978,0.,0.228856762039213));
#7482=DIRECTION('',(-0.973460108308978,0.,-0.228856762039213));
#7483=DIRECTION('',(0.,1.,0.));
#7484=DIRECTION('center_axis',(0.718125543087909,0.,0.695913575355946));
#7485=DIRECTION('ref_axis',(0.695913575355946,0.,-0.718125543087909));
#7486=DIRECTION('',(-0.695913575355946,0.,0.718125543087909));
#7487=DIRECTION('',(0.695913575355946,0.,-0.718125543087909));
#7488=DIRECTION('',(0.,1.,0.));
#7489=DIRECTION('center_axis',(0.473008672652493,0.,-0.881057770861552));
#7490=DIRECTION('ref_axis',(-0.881057770861552,0.,-0.473008672652493));
#7491=DIRECTION('',(0.881057770861552,0.,0.473008672652493));
#7492=DIRECTION('',(-0.881057770861552,0.,-0.473008672652493));
#7493=DIRECTION('',(0.,1.,0.));
#7494=DIRECTION('center_axis',(0.513540321538969,0.,0.858065462627213));
#7495=DIRECTION('ref_axis',(0.858065462627213,0.,-0.513540321538969));
#7496=DIRECTION('',(-0.858065462627213,0.,0.513540321538969));
#7497=DIRECTION('',(0.858065462627213,0.,-0.513540321538969));
#7498=DIRECTION('',(0.,1.,0.));
#7499=DIRECTION('center_axis',(0.684925823908296,0.,-0.728612802346721));
#7500=DIRECTION('ref_axis',(-0.728612802346721,0.,-0.684925823908296));
#7501=DIRECTION('',(0.728612802346721,0.,0.684925823908296));
#7502=DIRECTION('',(-0.728612802346721,0.,-0.684925823908296));
#7503=DIRECTION('',(0.,1.,0.));
#7504=DIRECTION('center_axis',(0.27395817574266,0.,0.961741606640658));
#7505=DIRECTION('ref_axis',(0.961741606640658,0.,-0.27395817574266));
#7506=DIRECTION('',(-0.961741606640658,0.,0.27395817574266));
#7507=DIRECTION('',(0.961741606640658,0.,-0.27395817574266));
#7508=DIRECTION('',(0.,1.,0.));
#7509=DIRECTION('center_axis',(0.850166412158193,0.,-0.526514075441546));
#7510=DIRECTION('ref_axis',(-0.526514075441546,0.,-0.850166412158193));
#7511=DIRECTION('',(0.526514075441546,0.,0.850166412158193));
#7512=DIRECTION('',(-0.526514075441546,0.,-0.850166412158193));
#7513=DIRECTION('center_axis',(0.,1.,0.));
#7514=DIRECTION('ref_axis',(0.,0.,1.));
#7515=DIRECTION('center_axis',(0.,1.,0.));
#7516=DIRECTION('ref_axis',(1.,0.,0.));
#10673=CARTESIAN_POINT('',(0.,0.,0.));
#10674=CARTESIAN_POINT('Origin',(0.,-2.4,7.52));
#10675=CARTESIAN_POINT('',(0.172988438920056,-2.51905880899792,7.52));
#10676=CARTESIAN_POINT('',(0.172988438920056,-2.28094119100208,7.52));
#10677=CARTESIAN_POINT('',(0.172988438920056,-3.6,7.52));
#10678=CARTESIAN_POINT('Origin',(0.,-2.4,7.52));
#10679=CARTESIAN_POINT('Origin',(0.,-2.4,7.52));
#10680=CARTESIAN_POINT('',(-0.172988438920056,-2.51905880899792,7.52));
#10681=CARTESIAN_POINT('Ctrl Pts',(-0.172988438920056,-2.51905880899792,
7.52));
#10682=CARTESIAN_POINT('Ctrl Pts',(-0.165594865311314,-2.52980142239529,
7.52129192197638));
#10683=CARTESIAN_POINT('Ctrl Pts',(-0.157297138725606,-2.53968770937274,
7.52265394943905));
#10684=CARTESIAN_POINT('Ctrl Pts',(-0.129892073845076,-2.56709277425327,
7.5267480843909));
#10685=CARTESIAN_POINT('Ctrl Pts',(-0.106330167759285,-2.58324205633295,
7.52969589327638));
#10686=CARTESIAN_POINT('Ctrl Pts',(-0.0546129046324105,-2.60469779396491,
7.53385029472357));
#10687=CARTESIAN_POINT('Ctrl Pts',(-0.0264512308298517,-2.61,7.535));
#10688=CARTESIAN_POINT('Ctrl Pts',(0.0264512308298516,-2.61,7.535));
#10689=CARTESIAN_POINT('Ctrl Pts',(0.0546129046324104,-2.60469779396491,
7.53385029472357));
#10690=CARTESIAN_POINT('Ctrl Pts',(0.106330167759284,-2.58324205633295,
7.52969589327638));
#10691=CARTESIAN_POINT('Ctrl Pts',(0.129892073845076,-2.56709277425327,
7.5267480843909));
#10692=CARTESIAN_POINT('Ctrl Pts',(0.157297138725606,-2.53968770937274,
7.52265394943905));
#10693=CARTESIAN_POINT('Ctrl Pts',(0.165594865311314,-2.52980142239529,
7.52129192197638));
#10694=CARTESIAN_POINT('Ctrl Pts',(0.172988438920056,-2.51905880899792,
7.52));
#10695=CARTESIAN_POINT('',(-0.21,-2.4,7.52));
#10696=CARTESIAN_POINT('Origin',(0.,-2.4,7.52));
#10697=CARTESIAN_POINT('',(-0.21,-2.4,8.11615888233178));
#10698=CARTESIAN_POINT('',(-0.21,-2.4,7.52));
#10699=CARTESIAN_POINT('',(0.21,-2.4,8.11615888233178));
#10700=CARTESIAN_POINT('Ctrl Pts',(0.21,-2.4,8.11615888233178));
#10701=CARTESIAN_POINT('Ctrl Pts',(0.21,-2.42640093420375,8.11615888233178));
#10702=CARTESIAN_POINT('Ctrl Pts',(0.20471752266132,-2.45454055536511,8.11688606295397));
#10703=CARTESIAN_POINT('Ctrl Pts',(0.183276841782292,-2.5062710523005,8.11950502964782));
#10704=CARTESIAN_POINT('Ctrl Pts',(0.167120287247804,-2.52986456085055,
8.12135816887013));
#10705=CARTESIAN_POINT('Ctrl Pts',(0.129864750292352,-2.567120097806,8.12483075953278));
#10706=CARTESIAN_POINT('Ctrl Pts',(0.106271159541076,-2.58327680083123,
8.12667690933009));
#10707=CARTESIAN_POINT('Ctrl Pts',(0.0545403836274688,-2.6047175903444,
8.12927985626981));
#10708=CARTESIAN_POINT('Ctrl Pts',(0.0264006657112965,-2.61,8.13));
#10709=CARTESIAN_POINT('Ctrl Pts',(-0.0264006657112964,-2.61,8.13));
#10710=CARTESIAN_POINT('Ctrl Pts',(-0.0545403836274688,-2.6047175903444,
8.12927985626981));
#10711=CARTESIAN_POINT('Ctrl Pts',(-0.106271159541076,-2.58327680083123,
8.12667690933009));
#10712=CARTESIAN_POINT('Ctrl Pts',(-0.129864750292352,-2.567120097806,8.12483075953278));
#10713=CARTESIAN_POINT('Ctrl Pts',(-0.167120287247804,-2.52986456085055,
8.12135816887013));
#10714=CARTESIAN_POINT('Ctrl Pts',(-0.183276841782292,-2.5062710523005,
8.11950502964782));
#10715=CARTESIAN_POINT('Ctrl Pts',(-0.20471752266132,-2.45454055536511,
8.11688606295397));
#10716=CARTESIAN_POINT('Ctrl Pts',(-0.21,-2.42640093420375,8.11615888233178));
#10717=CARTESIAN_POINT('Ctrl Pts',(-0.21,-2.4,8.11615888233178));
#10718=CARTESIAN_POINT('Ctrl Pts',(-0.21,-2.4,8.11615888233178));
#10719=CARTESIAN_POINT('Ctrl Pts',(-0.21,-2.37359906579625,8.11615888233178));
#10720=CARTESIAN_POINT('Ctrl Pts',(-0.20471752266132,-2.34545944463489,
8.11688606295397));
#10721=CARTESIAN_POINT('Ctrl Pts',(-0.183276841782292,-2.2937289476995,
8.11950502964782));
#10722=CARTESIAN_POINT('Ctrl Pts',(-0.167120287247804,-2.27013543914945,
8.12135816887013));
#10723=CARTESIAN_POINT('Ctrl Pts',(-0.129864750292352,-2.232879902194,8.12483075953278));
#10724=CARTESIAN_POINT('Ctrl Pts',(-0.106271159541076,-2.21672319916877,
8.12667690933009));
#10725=CARTESIAN_POINT('Ctrl Pts',(-0.0545403836274688,-2.1952824096556,
8.12927985626981));
#10726=CARTESIAN_POINT('Ctrl Pts',(-0.0264006657112965,-2.19,8.13));
#10727=CARTESIAN_POINT('Ctrl Pts',(0.0264006657112965,-2.19,8.13));
#10728=CARTESIAN_POINT('Ctrl Pts',(0.0545403836274689,-2.1952824096556,
8.12927985626981));
#10729=CARTESIAN_POINT('Ctrl Pts',(0.106271159541076,-2.21672319916877,
8.12667690933009));
#10730=CARTESIAN_POINT('Ctrl Pts',(0.129864750292352,-2.232879902194,8.12483075953278));
#10731=CARTESIAN_POINT('Ctrl Pts',(0.167120287247804,-2.27013543914945,
8.12135816887013));
#10732=CARTESIAN_POINT('Ctrl Pts',(0.183276841782292,-2.2937289476995,8.11950502964782));
#10733=CARTESIAN_POINT('Ctrl Pts',(0.20471752266132,-2.34545944463489,8.11688606295397));
#10734=CARTESIAN_POINT('Ctrl Pts',(0.21,-2.37359906579625,8.11615888233178));
#10735=CARTESIAN_POINT('Ctrl Pts',(0.21,-2.4,8.11615888233178));
#10736=CARTESIAN_POINT('',(-0.172988438920056,-2.28094119100208,7.52));
#10737=CARTESIAN_POINT('Origin',(0.,-2.4,7.52));
#10738=CARTESIAN_POINT('Ctrl Pts',(0.172988438920056,-2.28094119100209,
7.52));
#10739=CARTESIAN_POINT('Ctrl Pts',(0.165594865311314,-2.27019857760471,
7.52129192197638));
#10740=CARTESIAN_POINT('Ctrl Pts',(0.157297138725606,-2.26031229062726,
7.52265394943905));
#10741=CARTESIAN_POINT('Ctrl Pts',(0.129892073845076,-2.23290722574673,
7.5267480843909));
#10742=CARTESIAN_POINT('Ctrl Pts',(0.106330167759284,-2.21675794366705,
7.52969589327638));
#10743=CARTESIAN_POINT('Ctrl Pts',(0.0546129046324104,-2.19530220603509,
7.53385029472357));
#10744=CARTESIAN_POINT('Ctrl Pts',(0.0264512308298516,-2.19,7.535));
#10745=CARTESIAN_POINT('Ctrl Pts',(-0.0264512308298516,-2.19,7.535));
#10746=CARTESIAN_POINT('Ctrl Pts',(-0.0546129046324104,-2.19530220603509,
7.53385029472357));
#10747=CARTESIAN_POINT('Ctrl Pts',(-0.106330167759284,-2.21675794366705,
7.52969589327638));
#10748=CARTESIAN_POINT('Ctrl Pts',(-0.129892073845076,-2.23290722574673,
7.5267480843909));
#10749=CARTESIAN_POINT('Ctrl Pts',(-0.157297138725606,-2.26031229062726,
7.52265394943905));
#10750=CARTESIAN_POINT('Ctrl Pts',(-0.165594865311315,-2.27019857760471,
7.52129192197638));
#10751=CARTESIAN_POINT('Ctrl Pts',(-0.172988438920056,-2.28094119100208,
7.52));
#10752=CARTESIAN_POINT('Origin',(0.,-2.4,7.52));
#10753=CARTESIAN_POINT('',(-0.172988438920056,-3.6,7.52));
#10754=CARTESIAN_POINT('Origin',(0.,-2.9,6.53));
#10755=CARTESIAN_POINT('',(-1.6,-1.9,6.53));
#10756=CARTESIAN_POINT('Origin',(0.,-1.9,6.53));
#10757=CARTESIAN_POINT('',(-1.6,-2.9,6.53));
#10758=CARTESIAN_POINT('',(-1.6,-2.9,6.53));
#10759=CARTESIAN_POINT('Origin',(0.,-2.9,6.53));
#10760=CARTESIAN_POINT('Origin',(0.,-1.9,6.53));
#10761=CARTESIAN_POINT('',(-1.005,-1.9,6.53));
#10762=CARTESIAN_POINT('Origin',(0.,-1.9,6.53));
#10763=CARTESIAN_POINT('Origin',(0.,-3.6,6.53));
#10764=CARTESIAN_POINT('',(-1.005,-3.5,6.53));
#10765=CARTESIAN_POINT('Origin',(0.,-3.5,6.53));
#10766=CARTESIAN_POINT('',(-1.005,-3.6,6.53));
#10767=CARTESIAN_POINT('Origin',(4.,-3.5,6.53));
#10768=CARTESIAN_POINT('',(4.49999314610979,-3.5,6.52214602235346));
#10769=CARTESIAN_POINT('',(4.,-3.5,6.53));
#10770=CARTESIAN_POINT('',(4.49999314610979,-3.5,6.52214602235346));
#10771=CARTESIAN_POINT('',(4.49999314610979,-2.9,6.52214602235346));
#10772=CARTESIAN_POINT('',(4.49999314610979,-3.5,6.52214602235346));
#10773=CARTESIAN_POINT('',(4.,-2.9,6.53));
#10774=CARTESIAN_POINT('',(4.49999314610979,-2.9,6.52214602235346));
#10775=CARTESIAN_POINT('',(4.,-3.5,6.53));
#10776=CARTESIAN_POINT('Origin',(4.34869235694598,-3.5,7.68709756919613));
#10777=CARTESIAN_POINT('',(4.34869235694598,-3.5,7.68709756919613));
#10778=CARTESIAN_POINT('',(4.,-3.5,6.53));
#10779=CARTESIAN_POINT('',(4.34869235694598,-2.9,7.68709756919613));
#10780=CARTESIAN_POINT('',(4.,-2.9,6.53));
#10781=CARTESIAN_POINT('',(4.34869235694598,-3.5,7.68709756919613));
#10782=CARTESIAN_POINT('Origin',(3.86370330515627,-3.5,7.56527618041008));
#10783=CARTESIAN_POINT('',(3.86370330515627,-3.5,7.56527618041008));
#10784=CARTESIAN_POINT('',(4.34869235694598,-3.5,7.68709756919613));
#10785=CARTESIAN_POINT('',(3.86370330515627,-2.9,7.56527618041008));
#10786=CARTESIAN_POINT('',(4.34869235694598,-2.9,7.68709756919613));
#10787=CARTESIAN_POINT('',(3.86370330515627,-3.5,7.56527618041008));
#10788=CARTESIAN_POINT('Origin',(3.90103537021021,-3.5,8.77319482889224));
#10789=CARTESIAN_POINT('',(3.90103537021021,-3.5,8.77319482889224));
#10790=CARTESIAN_POINT('',(3.86370330515627,-3.5,7.56527618041008));
#10791=CARTESIAN_POINT('',(3.90103537021021,-2.9,8.77319482889224));
#10792=CARTESIAN_POINT('',(3.86370330515627,-2.9,7.56527618041008));
#10793=CARTESIAN_POINT('',(3.90103537021021,-3.5,8.77319482889224));
#10794=CARTESIAN_POINT('Origin',(3.46410161513775,-3.5,8.53));
#10795=CARTESIAN_POINT('',(3.46410161513775,-3.5,8.53));
#10796=CARTESIAN_POINT('',(3.90103537021021,-3.5,8.77319482889224));
#10797=CARTESIAN_POINT('',(3.46410161513775,-2.9,8.53));
#10798=CARTESIAN_POINT('',(3.90103537021021,-2.9,8.77319482889224));
#10799=CARTESIAN_POINT('',(3.46410161513775,-3.5,8.53));
#10800=CARTESIAN_POINT('Origin',(3.18752926976038,-3.5,9.70642206805406));
#10801=CARTESIAN_POINT('',(3.18752926976038,-3.5,9.70642206805406));
#10802=CARTESIAN_POINT('',(3.46410161513775,-3.5,8.53));
#10803=CARTESIAN_POINT('',(3.18752926976038,-2.9,9.70642206805406));
#10804=CARTESIAN_POINT('',(3.46410161513775,-2.9,8.53));
#10805=CARTESIAN_POINT('',(3.18752926976038,-3.5,9.70642206805406));
#10806=CARTESIAN_POINT('Origin',(2.82842712474619,-3.5,9.35842712474619));
#10807=CARTESIAN_POINT('',(2.82842712474619,-3.5,9.35842712474619));
#10808=CARTESIAN_POINT('',(3.18752926976038,-3.5,9.70642206805406));
#10809=CARTESIAN_POINT('',(2.82842712474619,-2.9,9.35842712474619));
#10810=CARTESIAN_POINT('',(3.18752926976038,-2.9,9.70642206805406));
#10811=CARTESIAN_POINT('',(2.82842712474619,-3.5,9.35842712474619));
#10812=CARTESIAN_POINT('Origin',(2.25679831721756,-3.5,10.4231813925637));
#10813=CARTESIAN_POINT('',(2.25679831721756,-3.5,10.4231813925637));
#10814=CARTESIAN_POINT('',(2.82842712474619,-3.5,9.35842712474619));
#10815=CARTESIAN_POINT('',(2.25679831721756,-2.9,10.4231813925637));
#10816=CARTESIAN_POINT('',(2.82842712474619,-2.9,9.35842712474619));
#10817=CARTESIAN_POINT('',(2.25679831721756,-3.5,10.4231813925637));
#10818=CARTESIAN_POINT('Origin',(2.,-3.5,9.99410161513775));
#10819=CARTESIAN_POINT('',(2.,-3.5,9.99410161513775));
#10820=CARTESIAN_POINT('',(2.25679831721756,-3.5,10.4231813925637));
#10821=CARTESIAN_POINT('',(2.,-2.9,9.99410161513775));
#10822=CARTESIAN_POINT('',(2.25679831721756,-2.9,10.4231813925637));
#10823=CARTESIAN_POINT('',(2.,-3.5,9.99410161513775));
#10824=CARTESIAN_POINT('Origin',(1.17227028889192,-3.5,10.8746268389565));
#10825=CARTESIAN_POINT('',(1.17227028889192,-3.5,10.8746268389565));
#10826=CARTESIAN_POINT('',(2.,-3.5,9.99410161513775));
#10827=CARTESIAN_POINT('',(1.17227028889192,-2.9,10.8746268389565));
#10828=CARTESIAN_POINT('',(2.,-2.9,9.99410161513775));
#10829=CARTESIAN_POINT('',(1.17227028889192,-3.5,10.8746268389565));
#10830=CARTESIAN_POINT('Origin',(1.03527618041008,-3.5,10.3937033051563));
#10831=CARTESIAN_POINT('',(1.03527618041008,-3.5,10.3937033051563));
#10832=CARTESIAN_POINT('',(1.17227028889192,-3.5,10.8746268389565));
#10833=CARTESIAN_POINT('',(1.03527618041008,-2.9,10.3937033051563));
#10834=CARTESIAN_POINT('',(1.17227028889192,-2.9,10.8746268389565));
#10835=CARTESIAN_POINT('',(1.03527618041008,-3.5,10.3937033051563));
#10836=CARTESIAN_POINT('Origin',(0.00785397764654228,-3.5,11.0299931461098));
#10837=CARTESIAN_POINT('',(0.00785397764654218,-3.5,11.0299931461098));
#10838=CARTESIAN_POINT('',(1.03527618041008,-3.5,10.3937033051563));
#10839=CARTESIAN_POINT('',(0.00785397764654228,-2.9,11.0299931461098));
#10840=CARTESIAN_POINT('',(1.03527618041008,-2.9,10.3937033051563));
#10841=CARTESIAN_POINT('',(0.00785397764654218,-3.5,11.0299931461098));
#10842=CARTESIAN_POINT('Origin',(2.4459601011273E-16,-3.5,10.53));
#10843=CARTESIAN_POINT('',(2.44929359829471E-16,-3.5,10.53));
#10844=CARTESIAN_POINT('',(0.00785397764654218,-3.5,11.0299931461098));
#10845=CARTESIAN_POINT('',(4.44089209850063E-16,-2.9,10.53));
#10846=CARTESIAN_POINT('',(0.00785397764654218,-2.9,11.0299931461098));
#10847=CARTESIAN_POINT('',(2.44929359829471E-16,-3.5,10.53));
#10848=CARTESIAN_POINT('Origin',(-1.15709756919613,-3.5,10.878692356946));
#10849=CARTESIAN_POINT('',(-1.15709756919613,-3.5,10.878692356946));
#10850=CARTESIAN_POINT('',(2.44929359829471E-16,-3.5,10.53));
#10851=CARTESIAN_POINT('',(-1.15709756919613,-2.9,10.878692356946));
#10852=CARTESIAN_POINT('',(2.44929359829471E-16,-2.9,10.53));
#10853=CARTESIAN_POINT('',(-1.15709756919613,-3.5,10.878692356946));
#10854=CARTESIAN_POINT('Origin',(-1.03527618041008,-3.5,10.3937033051563));
#10855=CARTESIAN_POINT('',(-1.03527618041008,-3.5,10.3937033051563));
#10856=CARTESIAN_POINT('',(-1.15709756919613,-3.5,10.878692356946));
#10857=CARTESIAN_POINT('',(-1.03527618041008,-2.9,10.3937033051563));
#10858=CARTESIAN_POINT('',(-1.15709756919613,-2.9,10.878692356946));
#10859=CARTESIAN_POINT('',(-1.03527618041008,-3.5,10.3937033051563));
#10860=CARTESIAN_POINT('Origin',(-2.24319482889224,-3.5,10.4310353702102));
#10861=CARTESIAN_POINT('',(-2.24319482889224,-3.5,10.4310353702102));
#10862=CARTESIAN_POINT('',(-1.03527618041008,-3.5,10.3937033051563));
#10863=CARTESIAN_POINT('',(-2.24319482889224,-2.9,10.4310353702102));
#10864=CARTESIAN_POINT('',(-1.03527618041008,-2.9,10.3937033051563));
#10865=CARTESIAN_POINT('',(-2.24319482889224,-3.5,10.4310353702102));
#10866=CARTESIAN_POINT('Origin',(-2.,-3.5,9.99410161513775));
#10867=CARTESIAN_POINT('',(-2.,-3.5,9.99410161513775));
#10868=CARTESIAN_POINT('',(-2.24319482889224,-3.5,10.4310353702102));
#10869=CARTESIAN_POINT('',(-2.,-2.9,9.99410161513775));
#10870=CARTESIAN_POINT('',(-2.24319482889224,-2.9,10.4310353702102));
#10871=CARTESIAN_POINT('',(-2.,-3.5,9.99410161513775));
#10872=CARTESIAN_POINT('Origin',(-3.17642206805406,-3.5,9.71752926976038));
#10873=CARTESIAN_POINT('',(-3.17642206805406,-3.5,9.71752926976038));
#10874=CARTESIAN_POINT('',(-2.,-3.5,9.99410161513775));
#10875=CARTESIAN_POINT('',(-3.17642206805406,-2.9,9.71752926976038));
#10876=CARTESIAN_POINT('',(-2.,-2.9,9.99410161513775));
#10877=CARTESIAN_POINT('',(-3.17642206805406,-3.5,9.71752926976038));
#10878=CARTESIAN_POINT('Origin',(-2.82842712474619,-3.5,9.35842712474619));
#10879=CARTESIAN_POINT('',(-2.82842712474619,-3.5,9.35842712474619));
#10880=CARTESIAN_POINT('',(-3.17642206805406,-3.5,9.71752926976038));
#10881=CARTESIAN_POINT('',(-2.82842712474619,-2.9,9.35842712474619));
#10882=CARTESIAN_POINT('',(-3.17642206805406,-2.9,9.71752926976038));
#10883=CARTESIAN_POINT('',(-2.82842712474619,-3.5,9.35842712474619));
#10884=CARTESIAN_POINT('Origin',(-3.89318139256367,-3.5,8.78679831721756));
#10885=CARTESIAN_POINT('',(-3.89318139256367,-3.5,8.78679831721756));
#10886=CARTESIAN_POINT('',(-2.82842712474619,-3.5,9.35842712474619));
#10887=CARTESIAN_POINT('',(-3.89318139256367,-2.9,8.78679831721756));
#10888=CARTESIAN_POINT('',(-2.82842712474619,-2.9,9.35842712474619));
#10889=CARTESIAN_POINT('',(-3.89318139256367,-3.5,8.78679831721756));
#10890=CARTESIAN_POINT('Origin',(-3.46410161513775,-3.5,8.53));
#10891=CARTESIAN_POINT('',(-3.46410161513775,-3.5,8.53));
#10892=CARTESIAN_POINT('',(-3.89318139256367,-3.5,8.78679831721756));
#10893=CARTESIAN_POINT('',(-3.46410161513775,-2.9,8.53));
#10894=CARTESIAN_POINT('',(-3.89318139256367,-2.9,8.78679831721756));
#10895=CARTESIAN_POINT('',(-3.46410161513775,-3.5,8.53));
#10896=CARTESIAN_POINT('Origin',(-4.34462683895651,-3.5,7.70227028889192));
#10897=CARTESIAN_POINT('',(-4.34462683895651,-3.5,7.70227028889192));
#10898=CARTESIAN_POINT('',(-3.46410161513775,-3.5,8.53));
#10899=CARTESIAN_POINT('',(-4.34462683895651,-2.9,7.70227028889192));
#10900=CARTESIAN_POINT('',(-3.46410161513775,-2.9,8.53));
#10901=CARTESIAN_POINT('',(-4.34462683895651,-3.5,7.70227028889192));
#10902=CARTESIAN_POINT('Origin',(-3.86370330515627,-3.5,7.56527618041008));
#10903=CARTESIAN_POINT('',(-3.86370330515627,-3.5,7.56527618041008));
#10904=CARTESIAN_POINT('',(-4.34462683895651,-3.5,7.70227028889192));
#10905=CARTESIAN_POINT('',(-3.86370330515627,-2.9,7.56527618041008));
#10906=CARTESIAN_POINT('',(-4.34462683895651,-2.9,7.70227028889192));
#10907=CARTESIAN_POINT('',(-3.86370330515627,-3.5,7.56527618041008));
#10908=CARTESIAN_POINT('Origin',(-4.49999314610979,-3.5,6.53785397764654));
#10909=CARTESIAN_POINT('',(-4.49999314610979,-3.5,6.53785397764654));
#10910=CARTESIAN_POINT('',(-3.86370330515627,-3.5,7.56527618041008));
#10911=CARTESIAN_POINT('',(-4.49999314610979,-2.9,6.53785397764654));
#10912=CARTESIAN_POINT('',(-3.86370330515627,-2.9,7.56527618041008));
#10913=CARTESIAN_POINT('',(-4.49999314610979,-3.5,6.53785397764654));
#10914=CARTESIAN_POINT('Origin',(-4.,-3.5,6.53));
#10915=CARTESIAN_POINT('',(-4.,-3.5,6.53));
#10916=CARTESIAN_POINT('',(-4.49999314610979,-3.5,6.53785397764654));
#10917=CARTESIAN_POINT('',(-4.,-2.9,6.53));
#10918=CARTESIAN_POINT('',(-4.49999314610979,-2.9,6.53785397764654));
#10919=CARTESIAN_POINT('',(-4.,-3.5,6.53));
#10920=CARTESIAN_POINT('Origin',(-4.34869235694598,-3.5,5.37290243080387));
#10921=CARTESIAN_POINT('',(-4.34869235694598,-3.5,5.37290243080387));
#10922=CARTESIAN_POINT('',(-4.,-3.5,6.53));
#10923=CARTESIAN_POINT('',(-4.34869235694598,-2.9,5.37290243080387));
#10924=CARTESIAN_POINT('',(-4.,-2.9,6.53));
#10925=CARTESIAN_POINT('',(-4.34869235694598,-3.5,5.37290243080387));
#10926=CARTESIAN_POINT('Origin',(-3.86370330515627,-3.5,5.49472381958992));
#10927=CARTESIAN_POINT('',(-3.86370330515627,-3.5,5.49472381958992));
#10928=CARTESIAN_POINT('',(-4.34869235694598,-3.5,5.37290243080387));
#10929=CARTESIAN_POINT('',(-3.86370330515627,-2.9,5.49472381958992));
#10930=CARTESIAN_POINT('',(-4.34869235694598,-2.9,5.37290243080387));
#10931=CARTESIAN_POINT('',(-3.86370330515627,-3.5,5.49472381958992));
#10932=CARTESIAN_POINT('Origin',(-3.90103537021021,-3.5,4.28680517110776));
#10933=CARTESIAN_POINT('',(-3.90103537021021,-3.5,4.28680517110776));
#10934=CARTESIAN_POINT('',(-3.86370330515627,-3.5,5.49472381958992));
#10935=CARTESIAN_POINT('',(-3.90103537021021,-2.9,4.28680517110776));
#10936=CARTESIAN_POINT('',(-3.86370330515627,-2.9,5.49472381958992));
#10937=CARTESIAN_POINT('',(-3.90103537021021,-3.5,4.28680517110776));
#10938=CARTESIAN_POINT('Origin',(-3.46410161513775,-3.5,4.53));
#10939=CARTESIAN_POINT('',(-3.46410161513775,-3.5,4.53));
#10940=CARTESIAN_POINT('',(-3.90103537021021,-3.5,4.28680517110776));
#10941=CARTESIAN_POINT('',(-3.46410161513775,-2.9,4.53));
#10942=CARTESIAN_POINT('',(-3.90103537021021,-2.9,4.28680517110776));
#10943=CARTESIAN_POINT('',(-3.46410161513775,-3.5,4.53));
#10944=CARTESIAN_POINT('Origin',(-3.18752926976038,-3.5,3.35357793194594));
#10945=CARTESIAN_POINT('',(-3.18752926976038,-3.5,3.35357793194594));
#10946=CARTESIAN_POINT('',(-3.46410161513775,-3.5,4.53));
#10947=CARTESIAN_POINT('',(-3.18752926976038,-2.9,3.35357793194594));
#10948=CARTESIAN_POINT('',(-3.46410161513775,-2.9,4.53));
#10949=CARTESIAN_POINT('',(-3.18752926976038,-3.5,3.35357793194594));
#10950=CARTESIAN_POINT('Origin',(-2.82842712474619,-3.5,3.70157287525381));
#10951=CARTESIAN_POINT('',(-2.82842712474619,-3.5,3.70157287525381));
#10952=CARTESIAN_POINT('',(-3.18752926976038,-3.5,3.35357793194594));
#10953=CARTESIAN_POINT('',(-2.82842712474619,-2.9,3.70157287525381));
#10954=CARTESIAN_POINT('',(-3.18752926976038,-2.9,3.35357793194594));
#10955=CARTESIAN_POINT('',(-2.82842712474619,-3.5,3.70157287525381));
#10956=CARTESIAN_POINT('Origin',(-2.25679831721756,-3.5,2.63681860743633));
#10957=CARTESIAN_POINT('',(-2.25679831721756,-3.5,2.63681860743633));
#10958=CARTESIAN_POINT('',(-2.82842712474619,-3.5,3.70157287525381));
#10959=CARTESIAN_POINT('',(-2.25679831721756,-2.9,2.63681860743633));
#10960=CARTESIAN_POINT('',(-2.82842712474619,-2.9,3.70157287525381));
#10961=CARTESIAN_POINT('',(-2.25679831721756,-3.5,2.63681860743633));
#10962=CARTESIAN_POINT('Origin',(-2.,-3.5,3.06589838486225));
#10963=CARTESIAN_POINT('',(-2.,-3.5,3.06589838486225));
#10964=CARTESIAN_POINT('',(-2.25679831721756,-3.5,2.63681860743633));
#10965=CARTESIAN_POINT('',(-2.,-2.9,3.06589838486225));
#10966=CARTESIAN_POINT('',(-2.25679831721756,-2.9,2.63681860743633));
#10967=CARTESIAN_POINT('',(-2.,-3.5,3.06589838486225));
#10968=CARTESIAN_POINT('Origin',(-1.17227028889192,-3.5,2.18537316104349));
#10969=CARTESIAN_POINT('',(-1.17227028889192,-3.5,2.18537316104349));
#10970=CARTESIAN_POINT('',(-2.,-3.5,3.06589838486225));
#10971=CARTESIAN_POINT('',(-1.17227028889192,-2.9,2.18537316104349));
#10972=CARTESIAN_POINT('',(-2.,-2.9,3.06589838486225));
#10973=CARTESIAN_POINT('',(-1.17227028889192,-3.5,2.18537316104349));
#10974=CARTESIAN_POINT('Origin',(-1.03527618041008,-3.5,2.66629669484373));
#10975=CARTESIAN_POINT('',(-1.03527618041008,-3.5,2.66629669484373));
#10976=CARTESIAN_POINT('',(-1.17227028889192,-3.5,2.18537316104349));
#10977=CARTESIAN_POINT('',(-1.03527618041008,-2.9,2.66629669484373));
#10978=CARTESIAN_POINT('',(-1.17227028889192,-2.9,2.18537316104349));
#10979=CARTESIAN_POINT('',(-1.03527618041008,-3.5,2.66629669484373));
#10980=CARTESIAN_POINT('Origin',(-0.00785397764654272,-3.5,2.03000685389021));
#10981=CARTESIAN_POINT('',(-0.00785397764654273,-3.5,2.03000685389021));
#10982=CARTESIAN_POINT('',(-1.03527618041008,-3.5,2.66629669484373));
#10983=CARTESIAN_POINT('',(-0.00785397764654272,-2.9,2.03000685389021));
#10984=CARTESIAN_POINT('',(-1.03527618041008,-2.9,2.66629669484373));
#10985=CARTESIAN_POINT('',(-0.00785397764654273,-3.5,2.03000685389021));
#10986=CARTESIAN_POINT('Origin',(-7.35522753814166E-16,-3.5,2.53));
#10987=CARTESIAN_POINT('',(-7.34788079488412E-16,-3.5,2.53));
#10988=CARTESIAN_POINT('',(-0.00785397764654273,-3.5,2.03000685389021));
#10989=CARTESIAN_POINT('',(-8.88178419700125E-16,-2.9,2.53));
#10990=CARTESIAN_POINT('',(-0.00785397764654273,-2.9,2.03000685389021));
#10991=CARTESIAN_POINT('',(-7.34788079488412E-16,-3.5,2.53));
#10992=CARTESIAN_POINT('Origin',(1.15709756919613,-3.5,2.18130764305402));
#10993=CARTESIAN_POINT('',(1.15709756919613,-3.5,2.18130764305402));
#10994=CARTESIAN_POINT('',(-7.34788079488412E-16,-3.5,2.53));
#10995=CARTESIAN_POINT('',(1.15709756919613,-2.9,2.18130764305402));
#10996=CARTESIAN_POINT('',(-7.34788079488412E-16,-2.9,2.53));
#10997=CARTESIAN_POINT('',(1.15709756919613,-3.5,2.18130764305402));
#10998=CARTESIAN_POINT('Origin',(1.03527618041008,-3.5,2.66629669484373));
#10999=CARTESIAN_POINT('',(1.03527618041008,-3.5,2.66629669484373));
#11000=CARTESIAN_POINT('',(1.15709756919613,-3.5,2.18130764305402));
#11001=CARTESIAN_POINT('',(1.03527618041008,-2.9,2.66629669484373));
#11002=CARTESIAN_POINT('',(1.15709756919613,-2.9,2.18130764305402));
#11003=CARTESIAN_POINT('',(1.03527618041008,-3.5,2.66629669484373));
#11004=CARTESIAN_POINT('Origin',(2.24319482889223,-3.5,2.62896462978979));
#11005=CARTESIAN_POINT('',(2.24319482889223,-3.5,2.62896462978979));
#11006=CARTESIAN_POINT('',(1.03527618041008,-3.5,2.66629669484373));
#11007=CARTESIAN_POINT('',(2.24319482889223,-2.9,2.62896462978979));
#11008=CARTESIAN_POINT('',(1.03527618041008,-2.9,2.66629669484373));
#11009=CARTESIAN_POINT('',(2.24319482889223,-3.5,2.62896462978979));
#11010=CARTESIAN_POINT('Origin',(2.,-3.5,3.06589838486225));
#11011=CARTESIAN_POINT('',(2.,-3.5,3.06589838486225));
#11012=CARTESIAN_POINT('',(2.24319482889223,-3.5,2.62896462978979));
#11013=CARTESIAN_POINT('',(2.,-2.9,3.06589838486225));
#11014=CARTESIAN_POINT('',(2.24319482889223,-2.9,2.62896462978979));
#11015=CARTESIAN_POINT('',(2.,-3.5,3.06589838486225));
#11016=CARTESIAN_POINT('Origin',(3.17642206805406,-3.5,3.34247073023962));
#11017=CARTESIAN_POINT('',(3.17642206805406,-3.5,3.34247073023962));
#11018=CARTESIAN_POINT('',(2.,-3.5,3.06589838486225));
#11019=CARTESIAN_POINT('',(3.17642206805406,-2.9,3.34247073023962));
#11020=CARTESIAN_POINT('',(2.,-2.9,3.06589838486225));
#11021=CARTESIAN_POINT('',(3.17642206805406,-3.5,3.34247073023962));
#11022=CARTESIAN_POINT('Origin',(2.82842712474619,-3.5,3.70157287525381));
#11023=CARTESIAN_POINT('',(2.82842712474619,-3.5,3.70157287525381));
#11024=CARTESIAN_POINT('',(3.17642206805406,-3.5,3.34247073023962));
#11025=CARTESIAN_POINT('',(2.82842712474619,-2.9,3.70157287525381));
#11026=CARTESIAN_POINT('',(3.17642206805406,-2.9,3.34247073023962));
#11027=CARTESIAN_POINT('',(2.82842712474619,-3.5,3.70157287525381));
#11028=CARTESIAN_POINT('Origin',(3.89318139256367,-3.5,4.27320168278244));
#11029=CARTESIAN_POINT('',(3.89318139256367,-3.5,4.27320168278244));
#11030=CARTESIAN_POINT('',(2.82842712474619,-3.5,3.70157287525381));
#11031=CARTESIAN_POINT('',(3.89318139256367,-2.9,4.27320168278244));
#11032=CARTESIAN_POINT('',(2.82842712474619,-2.9,3.70157287525381));
#11033=CARTESIAN_POINT('',(3.89318139256367,-3.5,4.27320168278244));
#11034=CARTESIAN_POINT('Origin',(3.46410161513775,-3.5,4.53));
#11035=CARTESIAN_POINT('',(3.46410161513775,-3.5,4.53));
#11036=CARTESIAN_POINT('',(3.89318139256367,-3.5,4.27320168278244));
#11037=CARTESIAN_POINT('',(3.46410161513775,-2.9,4.53));
#11038=CARTESIAN_POINT('',(3.89318139256367,-2.9,4.27320168278244));
#11039=CARTESIAN_POINT('',(3.46410161513775,-3.5,4.53));
#11040=CARTESIAN_POINT('Origin',(4.34462683895651,-3.5,5.35772971110808));
#11041=CARTESIAN_POINT('',(4.34462683895651,-3.5,5.35772971110808));
#11042=CARTESIAN_POINT('',(3.46410161513775,-3.5,4.53));
#11043=CARTESIAN_POINT('',(4.34462683895651,-2.9,5.35772971110808));
#11044=CARTESIAN_POINT('',(3.46410161513775,-2.9,4.53));
#11045=CARTESIAN_POINT('',(4.34462683895651,-3.5,5.35772971110808));
#11046=CARTESIAN_POINT('Origin',(3.86370330515627,-3.5,5.49472381958992));
#11047=CARTESIAN_POINT('',(3.86370330515627,-3.5,5.49472381958992));
#11048=CARTESIAN_POINT('',(4.34462683895651,-3.5,5.35772971110808));
#11049=CARTESIAN_POINT('',(3.86370330515627,-2.9,5.49472381958992));
#11050=CARTESIAN_POINT('',(4.34462683895651,-2.9,5.35772971110808));
#11051=CARTESIAN_POINT('',(3.86370330515627,-3.5,5.49472381958992));
#11052=CARTESIAN_POINT('Origin',(4.49999314610979,-3.5,6.52214602235346));
#11053=CARTESIAN_POINT('',(3.86370330515627,-3.5,5.49472381958992));
#11054=CARTESIAN_POINT('',(3.86370330515627,-2.9,5.49472381958992));
#11055=CARTESIAN_POINT('Origin',(0.,-2.9,6.53));
#11056=CARTESIAN_POINT('Origin',(0.,-3.5,6.53));
#11224=UNCERTAINTY_MEASURE_WITH_UNIT(LENGTH_MEASURE(0.001),#11259,
'DISTANCE_ACCURACY_VALUE',
'Maximum model space distance between geometric entities at asserted c
onnectivities');
#11228=UNCERTAINTY_MEASURE_WITH_UNIT(LENGTH_MEASURE(0.001),#11259,
'DISTANCE_ACCURACY_VALUE',
'Maximum model space distance between geometric entities at asserted c
onnectivities');
#11254=(
GEOMETRIC_REPRESENTATION_CONTEXT(3)
GLOBAL_UNCERTAINTY_ASSIGNED_CONTEXT((#11224))
GLOBAL_UNIT_ASSIGNED_CONTEXT((#11259,#11261,#11262))
REPRESENTATION_CONTEXT('','3D')
);
#11258=(
GEOMETRIC_REPRESENTATION_CONTEXT(3)
GLOBAL_UNCERTAINTY_ASSIGNED_CONTEXT((#11228))
GLOBAL_UNIT_ASSIGNED_CONTEXT((#11259,#11261,#11262))
REPRESENTATION_CONTEXT('','3D')
);
#11259=(
LENGTH_UNIT()
NAMED_UNIT(*)
SI_UNIT(.CENTI.,.METRE.)
);
#11261=(
NAMED_UNIT(*)
PLANE_ANGLE_UNIT()
SI_UNIT($,.RADIAN.)
);
#11262=(
NAMED_UNIT(*)
SI_UNIT($,.STERADIAN.)
SOLID_ANGLE_UNIT()
);
#11288=SHAPE_DEFINITION_REPRESENTATION(#11345,#11384);
#11345=PRODUCT_DEFINITION_SHAPE('',$,#11414);
#11384=SHAPE_REPRESENTATION('',(#5947),#11254);
#11388=PRODUCT_DEFINITION_CONTEXT('part definition',#11477,'design');
#11414=PRODUCT_DEFINITION('Ratchet wheel','Ratchet wheel',#11443,#11388);
#11443=PRODUCT_DEFINITION_FORMATION('',$,#11504);
#11477=APPLICATION_CONTEXT(
'Core Data for Automotive Mechanical Design Process');
#11478=PRODUCT_CONTEXT('part definition',#11477,'mechanical');
#11504=PRODUCT('Ratchet wheel','Ratchet wheel','Ratchet wheel',(#11478));
#11571=COLOUR_RGB('Sky Blue',0.24,0.69,0.87);
#11572=FILL_AREA_STYLE_COLOUR('',#11571);
#11573=FILL_AREA_STYLE('',(#11572));
#11574=SURFACE_STYLE_FILL_AREA(#11573);
#11575=SURFACE_SIDE_STYLE('',(#11574));
#11576=SURFACE_STYLE_USAGE(.BOTH.,#11575);
#11577=PRESENTATION_STYLE_ASSIGNMENT((#11576));
ENDSEC;
END-ISO-10303-21;
